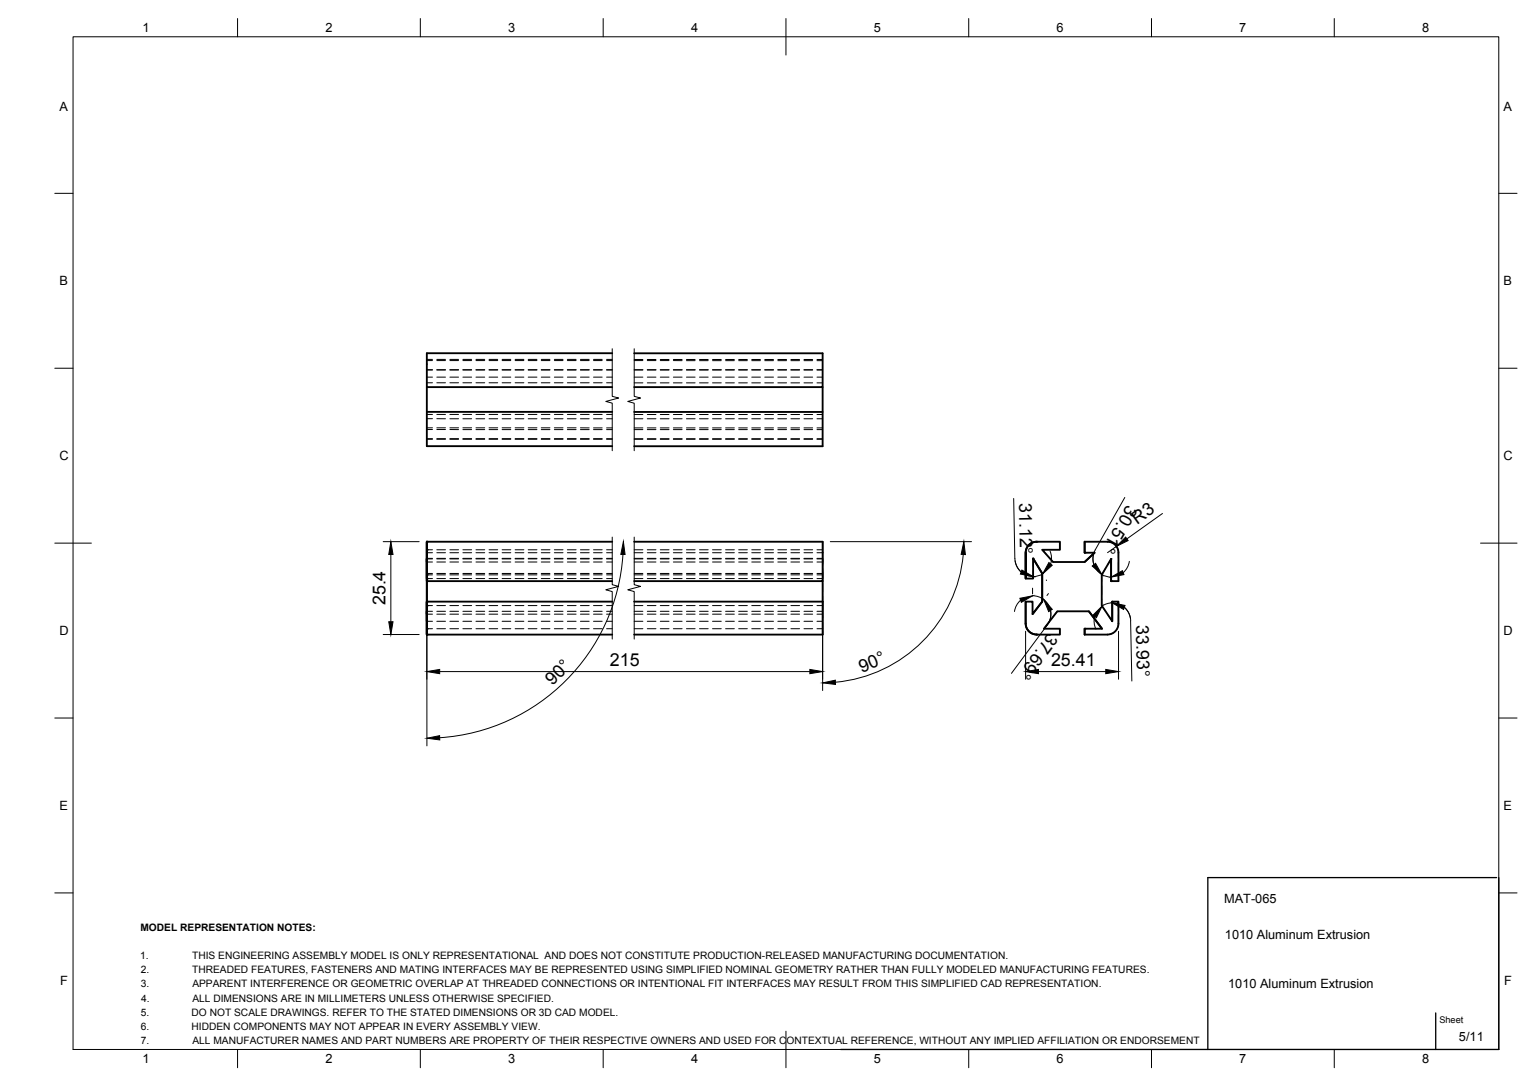
ISO-10303-21;
HEADER;
/* Generated by software containing ST-Developer
 * from STEP Tools, Inc. (www.steptools.com) 
 */

FILE_DESCRIPTION(
/* description */ (
'CAx-IF Rec.Pracs.---Representation and Presentation of Product Manufa
cturing Information (PMI)---4.0---2014-10-13'),
/* implementation_level */ '2;1');

FILE_NAME(
/* name */ '1010 Aluminum Extrusion.step',
/* time_stamp */ '2026-11-15T23:28:27-08:00',
/* author */ (''),
/* organization */ (''),
/* preprocessor_version */ 'ST-DEVELOPER v20.2',
/* originating_system */ 'Autodesk Translation Framework v15.17.0.0',
/* authorisation */ '');

FILE_SCHEMA (('AUTOMOTIVE_DESIGN { 1 0 10303 214 3 1 1 }'));
ENDSEC;

DATA;
#10=MECHANICAL_DESIGN_GEOMETRIC_PRESENTATION_REPRESENTATION('',(#194),#7756);
#176=SHAPE_REPRESENTATION_RELATIONSHIP('SRR','None',#7824,#185);
#185=ADVANCED_BREP_SHAPE_REPRESENTATION('',(#203),#7752);
#194=STYLED_ITEM('',(#7875),#203);
#203=MANIFOLD_SOLID_BREP('Body1',#4631);
#220=CYLINDRICAL_SURFACE('',#4850,0.003);
#221=CYLINDRICAL_SURFACE('',#4851,0.003);
#222=CYLINDRICAL_SURFACE('',#4852,0.003);
#223=CYLINDRICAL_SURFACE('',#4853,0.003);
#290=CIRCLE('',#4837,0.003);
#291=CIRCLE('',#4838,0.003);
#292=CIRCLE('',#4839,0.003);
#293=CIRCLE('',#4840,0.003);
#294=CIRCLE('',#4842,0.003);
#295=CIRCLE('',#4843,0.003);
#296=CIRCLE('',#4844,0.003);
#297=CIRCLE('',#4845,0.003);
#516=FACE_OUTER_BOUND('',#778,.T.);
#517=FACE_OUTER_BOUND('',#779,.T.);
#518=FACE_OUTER_BOUND('',#780,.T.);
#519=FACE_OUTER_BOUND('',#781,.T.);
#520=FACE_OUTER_BOUND('',#782,.T.);
#521=FACE_OUTER_BOUND('',#783,.T.);
#522=FACE_OUTER_BOUND('',#784,.T.);
#523=FACE_OUTER_BOUND('',#785,.T.);
#524=FACE_OUTER_BOUND('',#786,.T.);
#525=FACE_OUTER_BOUND('',#787,.T.);
#526=FACE_OUTER_BOUND('',#788,.T.);
#527=FACE_OUTER_BOUND('',#789,.T.);
#528=FACE_OUTER_BOUND('',#790,.T.);
#529=FACE_OUTER_BOUND('',#791,.T.);
#530=FACE_OUTER_BOUND('',#792,.T.);
#531=FACE_OUTER_BOUND('',#793,.T.);
#532=FACE_OUTER_BOUND('',#794,.T.);
#533=FACE_OUTER_BOUND('',#795,.T.);
#534=FACE_OUTER_BOUND('',#796,.T.);
#535=FACE_OUTER_BOUND('',#797,.T.);
#536=FACE_OUTER_BOUND('',#798,.T.);
#537=FACE_OUTER_BOUND('',#799,.T.);
#538=FACE_OUTER_BOUND('',#800,.T.);
#539=FACE_OUTER_BOUND('',#801,.T.);
#540=FACE_OUTER_BOUND('',#802,.T.);
#541=FACE_OUTER_BOUND('',#803,.T.);
#542=FACE_OUTER_BOUND('',#804,.T.);
#543=FACE_OUTER_BOUND('',#805,.T.);
#544=FACE_OUTER_BOUND('',#806,.T.);
#545=FACE_OUTER_BOUND('',#807,.T.);
#546=FACE_OUTER_BOUND('',#808,.T.);
#547=FACE_OUTER_BOUND('',#809,.T.);
#548=FACE_OUTER_BOUND('',#810,.T.);
#549=FACE_OUTER_BOUND('',#811,.T.);
#550=FACE_OUTER_BOUND('',#812,.T.);
#551=FACE_OUTER_BOUND('',#813,.T.);
#552=FACE_OUTER_BOUND('',#814,.T.);
#553=FACE_OUTER_BOUND('',#815,.T.);
#554=FACE_OUTER_BOUND('',#816,.T.);
#555=FACE_OUTER_BOUND('',#817,.T.);
#556=FACE_OUTER_BOUND('',#818,.T.);
#557=FACE_OUTER_BOUND('',#819,.T.);
#778=EDGE_LOOP('',(#3311,#3312,#3313,#3314));
#779=EDGE_LOOP('',(#3315,#3316,#3317,#3318));
#780=EDGE_LOOP('',(#3319,#3320,#3321,#3322));
#781=EDGE_LOOP('',(#3323,#3324,#3325,#3326));
#782=EDGE_LOOP('',(#3327,#3328,#3329,#3330,#3331,#3332,#3333,#3334,#3335,
#3336,#3337,#3338,#3339,#3340,#3341,#3342,#3343,#3344,#3345,#3346,#3347,
#3348,#3349,#3350,#3351,#3352,#3353,#3354,#3355,#3356,#3357,#3358,#3359,
#3360,#3361,#3362,#3363,#3364,#3365,#3366));
#783=EDGE_LOOP('',(#3367,#3368,#3369,#3370,#3371,#3372,#3373,#3374,#3375,
#3376,#3377,#3378,#3379,#3380,#3381,#3382,#3383,#3384,#3385,#3386,#3387,
#3388,#3389,#3390,#3391,#3392,#3393,#3394,#3395,#3396,#3397,#3398,#3399,
#3400,#3401,#3402,#3403,#3404,#3405,#3406));
#784=EDGE_LOOP('',(#3407,#3408,#3409,#3410));
#785=EDGE_LOOP('',(#3411,#3412,#3413,#3414));
#786=EDGE_LOOP('',(#3415,#3416,#3417,#3418));
#787=EDGE_LOOP('',(#3419,#3420,#3421,#3422));
#788=EDGE_LOOP('',(#3423,#3424,#3425,#3426));
#789=EDGE_LOOP('',(#3427,#3428,#3429,#3430));
#790=EDGE_LOOP('',(#3431,#3432,#3433,#3434));
#791=EDGE_LOOP('',(#3435,#3436,#3437,#3438));
#792=EDGE_LOOP('',(#3439,#3440,#3441,#3442));
#793=EDGE_LOOP('',(#3443,#3444,#3445,#3446));
#794=EDGE_LOOP('',(#3447,#3448,#3449,#3450));
#795=EDGE_LOOP('',(#3451,#3452,#3453,#3454));
#796=EDGE_LOOP('',(#3455,#3456,#3457,#3458));
#797=EDGE_LOOP('',(#3459,#3460,#3461,#3462));
#798=EDGE_LOOP('',(#3463,#3464,#3465,#3466));
#799=EDGE_LOOP('',(#3467,#3468,#3469,#3470));
#800=EDGE_LOOP('',(#3471,#3472,#3473,#3474));
#801=EDGE_LOOP('',(#3475,#3476,#3477,#3478));
#802=EDGE_LOOP('',(#3479,#3480,#3481,#3482));
#803=EDGE_LOOP('',(#3483,#3484,#3485,#3486));
#804=EDGE_LOOP('',(#3487,#3488,#3489,#3490));
#805=EDGE_LOOP('',(#3491,#3492,#3493,#3494));
#806=EDGE_LOOP('',(#3495,#3496,#3497,#3498));
#807=EDGE_LOOP('',(#3499,#3500,#3501,#3502));
#808=EDGE_LOOP('',(#3503,#3504,#3505,#3506));
#809=EDGE_LOOP('',(#3507,#3508,#3509,#3510));
#810=EDGE_LOOP('',(#3511,#3512,#3513,#3514));
#811=EDGE_LOOP('',(#3515,#3516,#3517,#3518));
#812=EDGE_LOOP('',(#3519,#3520,#3521,#3522));
#813=EDGE_LOOP('',(#3523,#3524,#3525,#3526));
#814=EDGE_LOOP('',(#3527,#3528,#3529,#3530));
#815=EDGE_LOOP('',(#3531,#3532,#3533,#3534));
#816=EDGE_LOOP('',(#3535,#3536,#3537,#3538));
#817=EDGE_LOOP('',(#3539,#3540,#3541,#3542));
#818=EDGE_LOOP('',(#3543,#3544,#3545,#3546));
#819=EDGE_LOOP('',(#3547,#3548,#3549,#3550));
#1125=LINE('',#6758,#1618);
#1126=LINE('',#6760,#1619);
#1127=LINE('',#6762,#1620);
#1128=LINE('',#6763,#1621);
#1129=LINE('',#6767,#1622);
#1130=LINE('',#6769,#1623);
#1131=LINE('',#6771,#1624);
#1132=LINE('',#6772,#1625);
#1133=LINE('',#6776,#1626);
#1134=LINE('',#6778,#1627);
#1135=LINE('',#6780,#1628);
#1136=LINE('',#6781,#1629);
#1137=LINE('',#6785,#1630);
#1138=LINE('',#6787,#1631);
#1139=LINE('',#6789,#1632);
#1140=LINE('',#6790,#1633);
#1141=LINE('',#6794,#1634);
#1142=LINE('',#6796,#1635);
#1143=LINE('',#6799,#1636);
#1144=LINE('',#6801,#1637);
#1145=LINE('',#6803,#1638);
#1146=LINE('',#6805,#1639);
#1147=LINE('',#6807,#1640);
#1148=LINE('',#6809,#1641);
#1149=LINE('',#6811,#1642);
#1150=LINE('',#6813,#1643);
#1151=LINE('',#6817,#1644);
#1152=LINE('',#6819,#1645);
#1153=LINE('',#6821,#1646);
#1154=LINE('',#6823,#1647);
#1155=LINE('',#6825,#1648);
#1156=LINE('',#6827,#1649);
#1157=LINE('',#6829,#1650);
#1158=LINE('',#6830,#1651);
#1159=LINE('',#6834,#1652);
#1160=LINE('',#6836,#1653);
#1161=LINE('',#6838,#1654);
#1162=LINE('',#6840,#1655);
#1163=LINE('',#6842,#1656);
#1164=LINE('',#6844,#1657);
#1165=LINE('',#6846,#1658);
#1166=LINE('',#6847,#1659);
#1167=LINE('',#6850,#1660);
#1168=LINE('',#6852,#1661);
#1169=LINE('',#6854,#1662);
#1170=LINE('',#6856,#1663);
#1171=LINE('',#6858,#1664);
#1172=LINE('',#6859,#1665);
#1173=LINE('',#6863,#1666);
#1174=LINE('',#6865,#1667);
#1175=LINE('',#6867,#1668);
#1176=LINE('',#6869,#1669);
#1177=LINE('',#6871,#1670);
#1178=LINE('',#6873,#1671);
#1179=LINE('',#6875,#1672);
#1180=LINE('',#6876,#1673);
#1181=LINE('',#6879,#1674);
#1182=LINE('',#6881,#1675);
#1183=LINE('',#6883,#1676);
#1184=LINE('',#6885,#1677);
#1185=LINE('',#6887,#1678);
#1186=LINE('',#6889,#1679);
#1187=LINE('',#6891,#1680);
#1188=LINE('',#6893,#1681);
#1189=LINE('',#6896,#1682);
#1190=LINE('',#6898,#1683);
#1191=LINE('',#6900,#1684);
#1192=LINE('',#6902,#1685);
#1193=LINE('',#6904,#1686);
#1194=LINE('',#6906,#1687);
#1195=LINE('',#6908,#1688);
#1196=LINE('',#6910,#1689);
#1197=LINE('',#6914,#1690);
#1198=LINE('',#6916,#1691);
#1199=LINE('',#6918,#1692);
#1200=LINE('',#6920,#1693);
#1201=LINE('',#6922,#1694);
#1202=LINE('',#6924,#1695);
#1203=LINE('',#6926,#1696);
#1204=LINE('',#6927,#1697);
#1205=LINE('',#6930,#1698);
#1206=LINE('',#6931,#1699);
#1207=LINE('',#6933,#1700);
#1208=LINE('',#6934,#1701);
#1209=LINE('',#6936,#1702);
#1210=LINE('',#6937,#1703);
#1211=LINE('',#6939,#1704);
#1212=LINE('',#6940,#1705);
#1213=LINE('',#6946,#1706);
#1214=LINE('',#6948,#1707);
#1215=LINE('',#6950,#1708);
#1216=LINE('',#6952,#1709);
#1217=LINE('',#6954,#1710);
#1218=LINE('',#6956,#1711);
#1219=LINE('',#6959,#1712);
#1220=LINE('',#6961,#1713);
#1221=LINE('',#6963,#1714);
#1222=LINE('',#6965,#1715);
#1223=LINE('',#6967,#1716);
#1224=LINE('',#6969,#1717);
#1225=LINE('',#6972,#1718);
#1226=LINE('',#6974,#1719);
#1227=LINE('',#6976,#1720);
#1228=LINE('',#6978,#1721);
#1229=LINE('',#6980,#1722);
#1230=LINE('',#6982,#1723);
#1231=LINE('',#6985,#1724);
#1232=LINE('',#6987,#1725);
#1233=LINE('',#6989,#1726);
#1234=LINE('',#6991,#1727);
#1235=LINE('',#6993,#1728);
#1236=LINE('',#6995,#1729);
#1618=VECTOR('',#5461,1.);
#1619=VECTOR('',#5462,1.);
#1620=VECTOR('',#5463,1.);
#1621=VECTOR('',#5464,1.);
#1622=VECTOR('',#5467,1.);
#1623=VECTOR('',#5468,1.);
#1624=VECTOR('',#5469,1.);
#1625=VECTOR('',#5470,1.);
#1626=VECTOR('',#5473,1.);
#1627=VECTOR('',#5474,1.);
#1628=VECTOR('',#5475,1.);
#1629=VECTOR('',#5476,1.);
#1630=VECTOR('',#5479,1.);
#1631=VECTOR('',#5480,1.);
#1632=VECTOR('',#5481,1.);
#1633=VECTOR('',#5482,1.);
#1634=VECTOR('',#5485,1.);
#1635=VECTOR('',#5486,1.);
#1636=VECTOR('',#5489,1.);
#1637=VECTOR('',#5490,1.);
#1638=VECTOR('',#5491,1.);
#1639=VECTOR('',#5492,1.);
#1640=VECTOR('',#5493,1.);
#1641=VECTOR('',#5494,1.);
#1642=VECTOR('',#5495,1.);
#1643=VECTOR('',#5496,1.);
#1644=VECTOR('',#5499,1.);
#1645=VECTOR('',#5500,1.);
#1646=VECTOR('',#5501,1.);
#1647=VECTOR('',#5502,1.);
#1648=VECTOR('',#5503,1.);
#1649=VECTOR('',#5504,1.);
#1650=VECTOR('',#5505,1.);
#1651=VECTOR('',#5506,1.);
#1652=VECTOR('',#5509,1.);
#1653=VECTOR('',#5510,1.);
#1654=VECTOR('',#5511,1.);
#1655=VECTOR('',#5512,1.);
#1656=VECTOR('',#5513,1.);
#1657=VECTOR('',#5514,1.);
#1658=VECTOR('',#5515,1.);
#1659=VECTOR('',#5516,1.);
#1660=VECTOR('',#5519,1.);
#1661=VECTOR('',#5520,1.);
#1662=VECTOR('',#5521,1.);
#1663=VECTOR('',#5522,1.);
#1664=VECTOR('',#5523,1.);
#1665=VECTOR('',#5524,1.);
#1666=VECTOR('',#5527,1.);
#1667=VECTOR('',#5528,1.);
#1668=VECTOR('',#5529,1.);
#1669=VECTOR('',#5530,1.);
#1670=VECTOR('',#5531,1.);
#1671=VECTOR('',#5532,1.);
#1672=VECTOR('',#5533,1.);
#1673=VECTOR('',#5534,1.);
#1674=VECTOR('',#5537,1.);
#1675=VECTOR('',#5538,1.);
#1676=VECTOR('',#5539,1.);
#1677=VECTOR('',#5540,1.);
#1678=VECTOR('',#5541,1.);
#1679=VECTOR('',#5542,1.);
#1680=VECTOR('',#5543,1.);
#1681=VECTOR('',#5544,1.);
#1682=VECTOR('',#5547,1.);
#1683=VECTOR('',#5548,1.);
#1684=VECTOR('',#5549,1.);
#1685=VECTOR('',#5550,1.);
#1686=VECTOR('',#5551,1.);
#1687=VECTOR('',#5552,1.);
#1688=VECTOR('',#5553,1.);
#1689=VECTOR('',#5554,1.);
#1690=VECTOR('',#5557,1.);
#1691=VECTOR('',#5558,1.);
#1692=VECTOR('',#5559,1.);
#1693=VECTOR('',#5560,1.);
#1694=VECTOR('',#5561,1.);
#1695=VECTOR('',#5562,1.);
#1696=VECTOR('',#5563,1.);
#1697=VECTOR('',#5564,1.);
#1698=VECTOR('',#5569,1.);
#1699=VECTOR('',#5570,1.);
#1700=VECTOR('',#5573,1.);
#1701=VECTOR('',#5574,1.);
#1702=VECTOR('',#5577,1.);
#1703=VECTOR('',#5578,1.);
#1704=VECTOR('',#5581,1.);
#1705=VECTOR('',#5582,1.);
#1706=VECTOR('',#5593,1.);
#1707=VECTOR('',#5596,1.);
#1708=VECTOR('',#5599,1.);
#1709=VECTOR('',#5602,1.);
#1710=VECTOR('',#5605,1.);
#1711=VECTOR('',#5608,1.);
#1712=VECTOR('',#5613,1.);
#1713=VECTOR('',#5616,1.);
#1714=VECTOR('',#5619,1.);
#1715=VECTOR('',#5622,1.);
#1716=VECTOR('',#5625,1.);
#1717=VECTOR('',#5628,1.);
#1718=VECTOR('',#5633,1.);
#1719=VECTOR('',#5636,1.);
#1720=VECTOR('',#5639,1.);
#1721=VECTOR('',#5642,1.);
#1722=VECTOR('',#5645,1.);
#1723=VECTOR('',#5648,1.);
#1724=VECTOR('',#5653,1.);
#1725=VECTOR('',#5656,1.);
#1726=VECTOR('',#5659,1.);
#1727=VECTOR('',#5662,1.);
#1728=VECTOR('',#5665,1.);
#1729=VECTOR('',#5668,1.);
#2084=VERTEX_POINT('',#6756);
#2085=VERTEX_POINT('',#6757);
#2086=VERTEX_POINT('',#6759);
#2087=VERTEX_POINT('',#6761);
#2088=VERTEX_POINT('',#6765);
#2089=VERTEX_POINT('',#6766);
#2090=VERTEX_POINT('',#6768);
#2091=VERTEX_POINT('',#6770);
#2092=VERTEX_POINT('',#6774);
#2093=VERTEX_POINT('',#6775);
#2094=VERTEX_POINT('',#6777);
#2095=VERTEX_POINT('',#6779);
#2096=VERTEX_POINT('',#6783);
#2097=VERTEX_POINT('',#6784);
#2098=VERTEX_POINT('',#6786);
#2099=VERTEX_POINT('',#6788);
#2100=VERTEX_POINT('',#6792);
#2101=VERTEX_POINT('',#6793);
#2102=VERTEX_POINT('',#6795);
#2103=VERTEX_POINT('',#6798);
#2104=VERTEX_POINT('',#6800);
#2105=VERTEX_POINT('',#6802);
#2106=VERTEX_POINT('',#6804);
#2107=VERTEX_POINT('',#6806);
#2108=VERTEX_POINT('',#6808);
#2109=VERTEX_POINT('',#6810);
#2110=VERTEX_POINT('',#6812);
#2111=VERTEX_POINT('',#6814);
#2112=VERTEX_POINT('',#6816);
#2113=VERTEX_POINT('',#6818);
#2114=VERTEX_POINT('',#6820);
#2115=VERTEX_POINT('',#6822);
#2116=VERTEX_POINT('',#6824);
#2117=VERTEX_POINT('',#6826);
#2118=VERTEX_POINT('',#6828);
#2119=VERTEX_POINT('',#6831);
#2120=VERTEX_POINT('',#6833);
#2121=VERTEX_POINT('',#6835);
#2122=VERTEX_POINT('',#6837);
#2123=VERTEX_POINT('',#6839);
#2124=VERTEX_POINT('',#6841);
#2125=VERTEX_POINT('',#6843);
#2126=VERTEX_POINT('',#6845);
#2127=VERTEX_POINT('',#6849);
#2128=VERTEX_POINT('',#6851);
#2129=VERTEX_POINT('',#6853);
#2130=VERTEX_POINT('',#6855);
#2131=VERTEX_POINT('',#6857);
#2132=VERTEX_POINT('',#6861);
#2133=VERTEX_POINT('',#6862);
#2134=VERTEX_POINT('',#6864);
#2135=VERTEX_POINT('',#6866);
#2136=VERTEX_POINT('',#6868);
#2137=VERTEX_POINT('',#6870);
#2138=VERTEX_POINT('',#6872);
#2139=VERTEX_POINT('',#6874);
#2140=VERTEX_POINT('',#6878);
#2141=VERTEX_POINT('',#6880);
#2142=VERTEX_POINT('',#6882);
#2143=VERTEX_POINT('',#6884);
#2144=VERTEX_POINT('',#6886);
#2145=VERTEX_POINT('',#6888);
#2146=VERTEX_POINT('',#6890);
#2147=VERTEX_POINT('',#6892);
#2148=VERTEX_POINT('',#6895);
#2149=VERTEX_POINT('',#6897);
#2150=VERTEX_POINT('',#6899);
#2151=VERTEX_POINT('',#6901);
#2152=VERTEX_POINT('',#6903);
#2153=VERTEX_POINT('',#6905);
#2154=VERTEX_POINT('',#6907);
#2155=VERTEX_POINT('',#6909);
#2156=VERTEX_POINT('',#6911);
#2157=VERTEX_POINT('',#6913);
#2158=VERTEX_POINT('',#6915);
#2159=VERTEX_POINT('',#6917);
#2160=VERTEX_POINT('',#6919);
#2161=VERTEX_POINT('',#6921);
#2162=VERTEX_POINT('',#6923);
#2163=VERTEX_POINT('',#6925);
#2539=EDGE_CURVE('',#2084,#2085,#1125,.T.);
#2540=EDGE_CURVE('',#2084,#2086,#1126,.T.);
#2541=EDGE_CURVE('',#2086,#2087,#1127,.T.);
#2542=EDGE_CURVE('',#2087,#2085,#1128,.T.);
#2543=EDGE_CURVE('',#2088,#2089,#1129,.T.);
#2544=EDGE_CURVE('',#2088,#2090,#1130,.T.);
#2545=EDGE_CURVE('',#2090,#2091,#1131,.F.);
#2546=EDGE_CURVE('',#2089,#2091,#1132,.T.);
#2547=EDGE_CURVE('',#2092,#2093,#1133,.T.);
#2548=EDGE_CURVE('',#2092,#2094,#1134,.T.);
#2549=EDGE_CURVE('',#2094,#2095,#1135,.F.);
#2550=EDGE_CURVE('',#2093,#2095,#1136,.T.);
#2551=EDGE_CURVE('',#2096,#2097,#1137,.T.);
#2552=EDGE_CURVE('',#2096,#2098,#1138,.T.);
#2553=EDGE_CURVE('',#2098,#2099,#1139,.T.);
#2554=EDGE_CURVE('',#2099,#2097,#1140,.T.);
#2555=EDGE_CURVE('',#2100,#2101,#1141,.T.);
#2556=EDGE_CURVE('',#2102,#2100,#1142,.T.);
#2557=EDGE_CURVE('',#2102,#2087,#290,.T.);
#2558=EDGE_CURVE('',#2103,#2086,#1143,.T.);
#2559=EDGE_CURVE('',#2104,#2103,#1144,.T.);
#2560=EDGE_CURVE('',#2105,#2104,#1145,.T.);
#2561=EDGE_CURVE('',#2106,#2105,#1146,.T.);
#2562=EDGE_CURVE('',#2107,#2106,#1147,.T.);
#2563=EDGE_CURVE('',#2108,#2107,#1148,.T.);
#2564=EDGE_CURVE('',#2109,#2108,#1149,.T.);
#2565=EDGE_CURVE('',#2110,#2109,#1150,.T.);
#2566=EDGE_CURVE('',#2110,#2111,#291,.T.);
#2567=EDGE_CURVE('',#2111,#2112,#1151,.T.);
#2568=EDGE_CURVE('',#2113,#2112,#1152,.T.);
#2569=EDGE_CURVE('',#2114,#2113,#1153,.T.);
#2570=EDGE_CURVE('',#2115,#2114,#1154,.T.);
#2571=EDGE_CURVE('',#2116,#2115,#1155,.T.);
#2572=EDGE_CURVE('',#2117,#2116,#1156,.T.);
#2573=EDGE_CURVE('',#2118,#2117,#1157,.T.);
#2574=EDGE_CURVE('',#2089,#2118,#1158,.T.);
#2575=EDGE_CURVE('',#2091,#2119,#292,.T.);
#2576=EDGE_CURVE('',#2119,#2120,#1159,.T.);
#2577=EDGE_CURVE('',#2120,#2121,#1160,.T.);
#2578=EDGE_CURVE('',#2121,#2122,#1161,.T.);
#2579=EDGE_CURVE('',#2122,#2123,#1162,.T.);
#2580=EDGE_CURVE('',#2123,#2124,#1163,.T.);
#2581=EDGE_CURVE('',#2124,#2125,#1164,.T.);
#2582=EDGE_CURVE('',#2125,#2126,#1165,.T.);
#2583=EDGE_CURVE('',#2126,#2093,#1166,.T.);
#2584=EDGE_CURVE('',#2095,#2099,#293,.T.);
#2585=EDGE_CURVE('',#2127,#2098,#1167,.T.);
#2586=EDGE_CURVE('',#2128,#2127,#1168,.T.);
#2587=EDGE_CURVE('',#2129,#2128,#1169,.T.);
#2588=EDGE_CURVE('',#2130,#2129,#1170,.T.);
#2589=EDGE_CURVE('',#2131,#2130,#1171,.T.);
#2590=EDGE_CURVE('',#2101,#2131,#1172,.T.);
#2591=EDGE_CURVE('',#2132,#2133,#1173,.T.);
#2592=EDGE_CURVE('',#2133,#2134,#1174,.T.);
#2593=EDGE_CURVE('',#2134,#2135,#1175,.T.);
#2594=EDGE_CURVE('',#2135,#2136,#1176,.T.);
#2595=EDGE_CURVE('',#2136,#2137,#1177,.T.);
#2596=EDGE_CURVE('',#2137,#2138,#1178,.T.);
#2597=EDGE_CURVE('',#2138,#2139,#1179,.T.);
#2598=EDGE_CURVE('',#2139,#2096,#1180,.T.);
#2599=EDGE_CURVE('',#2097,#2094,#294,.F.);
#2600=EDGE_CURVE('',#2140,#2092,#1181,.T.);
#2601=EDGE_CURVE('',#2141,#2140,#1182,.T.);
#2602=EDGE_CURVE('',#2142,#2141,#1183,.T.);
#2603=EDGE_CURVE('',#2143,#2142,#1184,.T.);
#2604=EDGE_CURVE('',#2144,#2143,#1185,.T.);
#2605=EDGE_CURVE('',#2145,#2144,#1186,.T.);
#2606=EDGE_CURVE('',#2146,#2145,#1187,.T.);
#2607=EDGE_CURVE('',#2147,#2146,#1188,.T.);
#2608=EDGE_CURVE('',#2147,#2090,#295,.F.);
#2609=EDGE_CURVE('',#2088,#2148,#1189,.T.);
#2610=EDGE_CURVE('',#2148,#2149,#1190,.T.);
#2611=EDGE_CURVE('',#2149,#2150,#1191,.T.);
#2612=EDGE_CURVE('',#2150,#2151,#1192,.T.);
#2613=EDGE_CURVE('',#2151,#2152,#1193,.T.);
#2614=EDGE_CURVE('',#2152,#2153,#1194,.T.);
#2615=EDGE_CURVE('',#2153,#2154,#1195,.T.);
#2616=EDGE_CURVE('',#2155,#2154,#1196,.T.);
#2617=EDGE_CURVE('',#2155,#2156,#296,.F.);
#2618=EDGE_CURVE('',#2156,#2157,#1197,.T.);
#2619=EDGE_CURVE('',#2157,#2158,#1198,.T.);
#2620=EDGE_CURVE('',#2158,#2159,#1199,.T.);
#2621=EDGE_CURVE('',#2159,#2160,#1200,.T.);
#2622=EDGE_CURVE('',#2160,#2161,#1201,.T.);
#2623=EDGE_CURVE('',#2161,#2162,#1202,.T.);
#2624=EDGE_CURVE('',#2162,#2163,#1203,.T.);
#2625=EDGE_CURVE('',#2163,#2084,#1204,.T.);
#2626=EDGE_CURVE('',#2085,#2132,#297,.F.);
#2627=EDGE_CURVE('',#2157,#2109,#1205,.T.);
#2628=EDGE_CURVE('',#2156,#2110,#1206,.F.);
#2629=EDGE_CURVE('',#2154,#2112,#1207,.T.);
#2630=EDGE_CURVE('',#2111,#2155,#1208,.T.);
#2631=EDGE_CURVE('',#2146,#2120,#1209,.T.);
#2632=EDGE_CURVE('',#2119,#2147,#1210,.T.);
#2633=EDGE_CURVE('',#2133,#2100,#1211,.T.);
#2634=EDGE_CURVE('',#2132,#2102,#1212,.F.);
#2635=EDGE_CURVE('',#2158,#2108,#1213,.T.);
#2636=EDGE_CURVE('',#2159,#2107,#1214,.T.);
#2637=EDGE_CURVE('',#2160,#2106,#1215,.T.);
#2638=EDGE_CURVE('',#2161,#2105,#1216,.T.);
#2639=EDGE_CURVE('',#2162,#2104,#1217,.T.);
#2640=EDGE_CURVE('',#2163,#2103,#1218,.T.);
#2641=EDGE_CURVE('',#2148,#2118,#1219,.T.);
#2642=EDGE_CURVE('',#2149,#2117,#1220,.T.);
#2643=EDGE_CURVE('',#2150,#2116,#1221,.T.);
#2644=EDGE_CURVE('',#2151,#2115,#1222,.T.);
#2645=EDGE_CURVE('',#2152,#2114,#1223,.T.);
#2646=EDGE_CURVE('',#2153,#2113,#1224,.T.);
#2647=EDGE_CURVE('',#2145,#2121,#1225,.T.);
#2648=EDGE_CURVE('',#2140,#2126,#1226,.T.);
#2649=EDGE_CURVE('',#2141,#2125,#1227,.T.);
#2650=EDGE_CURVE('',#2142,#2124,#1228,.T.);
#2651=EDGE_CURVE('',#2143,#2123,#1229,.T.);
#2652=EDGE_CURVE('',#2144,#2122,#1230,.T.);
#2653=EDGE_CURVE('',#2134,#2101,#1231,.T.);
#2654=EDGE_CURVE('',#2135,#2131,#1232,.T.);
#2655=EDGE_CURVE('',#2136,#2130,#1233,.T.);
#2656=EDGE_CURVE('',#2137,#2129,#1234,.T.);
#2657=EDGE_CURVE('',#2138,#2128,#1235,.T.);
#2658=EDGE_CURVE('',#2139,#2127,#1236,.T.);
#3311=ORIENTED_EDGE('',*,*,#2539,.F.);
#3312=ORIENTED_EDGE('',*,*,#2540,.T.);
#3313=ORIENTED_EDGE('',*,*,#2541,.T.);
#3314=ORIENTED_EDGE('',*,*,#2542,.T.);
#3315=ORIENTED_EDGE('',*,*,#2543,.F.);
#3316=ORIENTED_EDGE('',*,*,#2544,.T.);
#3317=ORIENTED_EDGE('',*,*,#2545,.T.);
#3318=ORIENTED_EDGE('',*,*,#2546,.F.);
#3319=ORIENTED_EDGE('',*,*,#2547,.F.);
#3320=ORIENTED_EDGE('',*,*,#2548,.T.);
#3321=ORIENTED_EDGE('',*,*,#2549,.T.);
#3322=ORIENTED_EDGE('',*,*,#2550,.F.);
#3323=ORIENTED_EDGE('',*,*,#2551,.F.);
#3324=ORIENTED_EDGE('',*,*,#2552,.T.);
#3325=ORIENTED_EDGE('',*,*,#2553,.T.);
#3326=ORIENTED_EDGE('',*,*,#2554,.T.);
#3327=ORIENTED_EDGE('',*,*,#2555,.F.);
#3328=ORIENTED_EDGE('',*,*,#2556,.F.);
#3329=ORIENTED_EDGE('',*,*,#2557,.T.);
#3330=ORIENTED_EDGE('',*,*,#2541,.F.);
#3331=ORIENTED_EDGE('',*,*,#2558,.F.);
#3332=ORIENTED_EDGE('',*,*,#2559,.F.);
#3333=ORIENTED_EDGE('',*,*,#2560,.F.);
#3334=ORIENTED_EDGE('',*,*,#2561,.F.);
#3335=ORIENTED_EDGE('',*,*,#2562,.F.);
#3336=ORIENTED_EDGE('',*,*,#2563,.F.);
#3337=ORIENTED_EDGE('',*,*,#2564,.F.);
#3338=ORIENTED_EDGE('',*,*,#2565,.F.);
#3339=ORIENTED_EDGE('',*,*,#2566,.T.);
#3340=ORIENTED_EDGE('',*,*,#2567,.T.);
#3341=ORIENTED_EDGE('',*,*,#2568,.F.);
#3342=ORIENTED_EDGE('',*,*,#2569,.F.);
#3343=ORIENTED_EDGE('',*,*,#2570,.F.);
#3344=ORIENTED_EDGE('',*,*,#2571,.F.);
#3345=ORIENTED_EDGE('',*,*,#2572,.F.);
#3346=ORIENTED_EDGE('',*,*,#2573,.F.);
#3347=ORIENTED_EDGE('',*,*,#2574,.F.);
#3348=ORIENTED_EDGE('',*,*,#2546,.T.);
#3349=ORIENTED_EDGE('',*,*,#2575,.T.);
#3350=ORIENTED_EDGE('',*,*,#2576,.T.);
#3351=ORIENTED_EDGE('',*,*,#2577,.T.);
#3352=ORIENTED_EDGE('',*,*,#2578,.T.);
#3353=ORIENTED_EDGE('',*,*,#2579,.T.);
#3354=ORIENTED_EDGE('',*,*,#2580,.T.);
#3355=ORIENTED_EDGE('',*,*,#2581,.T.);
#3356=ORIENTED_EDGE('',*,*,#2582,.T.);
#3357=ORIENTED_EDGE('',*,*,#2583,.T.);
#3358=ORIENTED_EDGE('',*,*,#2550,.T.);
#3359=ORIENTED_EDGE('',*,*,#2584,.T.);
#3360=ORIENTED_EDGE('',*,*,#2553,.F.);
#3361=ORIENTED_EDGE('',*,*,#2585,.F.);
#3362=ORIENTED_EDGE('',*,*,#2586,.F.);
#3363=ORIENTED_EDGE('',*,*,#2587,.F.);
#3364=ORIENTED_EDGE('',*,*,#2588,.F.);
#3365=ORIENTED_EDGE('',*,*,#2589,.F.);
#3366=ORIENTED_EDGE('',*,*,#2590,.F.);
#3367=ORIENTED_EDGE('',*,*,#2591,.T.);
#3368=ORIENTED_EDGE('',*,*,#2592,.T.);
#3369=ORIENTED_EDGE('',*,*,#2593,.T.);
#3370=ORIENTED_EDGE('',*,*,#2594,.T.);
#3371=ORIENTED_EDGE('',*,*,#2595,.T.);
#3372=ORIENTED_EDGE('',*,*,#2596,.T.);
#3373=ORIENTED_EDGE('',*,*,#2597,.T.);
#3374=ORIENTED_EDGE('',*,*,#2598,.T.);
#3375=ORIENTED_EDGE('',*,*,#2551,.T.);
#3376=ORIENTED_EDGE('',*,*,#2599,.T.);
#3377=ORIENTED_EDGE('',*,*,#2548,.F.);
#3378=ORIENTED_EDGE('',*,*,#2600,.F.);
#3379=ORIENTED_EDGE('',*,*,#2601,.F.);
#3380=ORIENTED_EDGE('',*,*,#2602,.F.);
#3381=ORIENTED_EDGE('',*,*,#2603,.F.);
#3382=ORIENTED_EDGE('',*,*,#2604,.F.);
#3383=ORIENTED_EDGE('',*,*,#2605,.F.);
#3384=ORIENTED_EDGE('',*,*,#2606,.F.);
#3385=ORIENTED_EDGE('',*,*,#2607,.F.);
#3386=ORIENTED_EDGE('',*,*,#2608,.T.);
#3387=ORIENTED_EDGE('',*,*,#2544,.F.);
#3388=ORIENTED_EDGE('',*,*,#2609,.T.);
#3389=ORIENTED_EDGE('',*,*,#2610,.T.);
#3390=ORIENTED_EDGE('',*,*,#2611,.T.);
#3391=ORIENTED_EDGE('',*,*,#2612,.T.);
#3392=ORIENTED_EDGE('',*,*,#2613,.T.);
#3393=ORIENTED_EDGE('',*,*,#2614,.T.);
#3394=ORIENTED_EDGE('',*,*,#2615,.T.);
#3395=ORIENTED_EDGE('',*,*,#2616,.F.);
#3396=ORIENTED_EDGE('',*,*,#2617,.T.);
#3397=ORIENTED_EDGE('',*,*,#2618,.T.);
#3398=ORIENTED_EDGE('',*,*,#2619,.T.);
#3399=ORIENTED_EDGE('',*,*,#2620,.T.);
#3400=ORIENTED_EDGE('',*,*,#2621,.T.);
#3401=ORIENTED_EDGE('',*,*,#2622,.T.);
#3402=ORIENTED_EDGE('',*,*,#2623,.T.);
#3403=ORIENTED_EDGE('',*,*,#2624,.T.);
#3404=ORIENTED_EDGE('',*,*,#2625,.T.);
#3405=ORIENTED_EDGE('',*,*,#2539,.T.);
#3406=ORIENTED_EDGE('',*,*,#2626,.T.);
#3407=ORIENTED_EDGE('',*,*,#2627,.F.);
#3408=ORIENTED_EDGE('',*,*,#2618,.F.);
#3409=ORIENTED_EDGE('',*,*,#2628,.T.);
#3410=ORIENTED_EDGE('',*,*,#2565,.T.);
#3411=ORIENTED_EDGE('',*,*,#2616,.T.);
#3412=ORIENTED_EDGE('',*,*,#2629,.T.);
#3413=ORIENTED_EDGE('',*,*,#2567,.F.);
#3414=ORIENTED_EDGE('',*,*,#2630,.T.);
#3415=ORIENTED_EDGE('',*,*,#2607,.T.);
#3416=ORIENTED_EDGE('',*,*,#2631,.T.);
#3417=ORIENTED_EDGE('',*,*,#2576,.F.);
#3418=ORIENTED_EDGE('',*,*,#2632,.T.);
#3419=ORIENTED_EDGE('',*,*,#2633,.F.);
#3420=ORIENTED_EDGE('',*,*,#2591,.F.);
#3421=ORIENTED_EDGE('',*,*,#2634,.T.);
#3422=ORIENTED_EDGE('',*,*,#2556,.T.);
#3423=ORIENTED_EDGE('',*,*,#2566,.F.);
#3424=ORIENTED_EDGE('',*,*,#2628,.F.);
#3425=ORIENTED_EDGE('',*,*,#2617,.F.);
#3426=ORIENTED_EDGE('',*,*,#2630,.F.);
#3427=ORIENTED_EDGE('',*,*,#2575,.F.);
#3428=ORIENTED_EDGE('',*,*,#2545,.F.);
#3429=ORIENTED_EDGE('',*,*,#2608,.F.);
#3430=ORIENTED_EDGE('',*,*,#2632,.F.);
#3431=ORIENTED_EDGE('',*,*,#2584,.F.);
#3432=ORIENTED_EDGE('',*,*,#2549,.F.);
#3433=ORIENTED_EDGE('',*,*,#2599,.F.);
#3434=ORIENTED_EDGE('',*,*,#2554,.F.);
#3435=ORIENTED_EDGE('',*,*,#2557,.F.);
#3436=ORIENTED_EDGE('',*,*,#2634,.F.);
#3437=ORIENTED_EDGE('',*,*,#2626,.F.);
#3438=ORIENTED_EDGE('',*,*,#2542,.F.);
#3439=ORIENTED_EDGE('',*,*,#2627,.T.);
#3440=ORIENTED_EDGE('',*,*,#2564,.T.);
#3441=ORIENTED_EDGE('',*,*,#2635,.F.);
#3442=ORIENTED_EDGE('',*,*,#2619,.F.);
#3443=ORIENTED_EDGE('',*,*,#2635,.T.);
#3444=ORIENTED_EDGE('',*,*,#2563,.T.);
#3445=ORIENTED_EDGE('',*,*,#2636,.F.);
#3446=ORIENTED_EDGE('',*,*,#2620,.F.);
#3447=ORIENTED_EDGE('',*,*,#2636,.T.);
#3448=ORIENTED_EDGE('',*,*,#2562,.T.);
#3449=ORIENTED_EDGE('',*,*,#2637,.F.);
#3450=ORIENTED_EDGE('',*,*,#2621,.F.);
#3451=ORIENTED_EDGE('',*,*,#2637,.T.);
#3452=ORIENTED_EDGE('',*,*,#2561,.T.);
#3453=ORIENTED_EDGE('',*,*,#2638,.F.);
#3454=ORIENTED_EDGE('',*,*,#2622,.F.);
#3455=ORIENTED_EDGE('',*,*,#2638,.T.);
#3456=ORIENTED_EDGE('',*,*,#2560,.T.);
#3457=ORIENTED_EDGE('',*,*,#2639,.F.);
#3458=ORIENTED_EDGE('',*,*,#2623,.F.);
#3459=ORIENTED_EDGE('',*,*,#2639,.T.);
#3460=ORIENTED_EDGE('',*,*,#2559,.T.);
#3461=ORIENTED_EDGE('',*,*,#2640,.F.);
#3462=ORIENTED_EDGE('',*,*,#2624,.F.);
#3463=ORIENTED_EDGE('',*,*,#2640,.T.);
#3464=ORIENTED_EDGE('',*,*,#2558,.T.);
#3465=ORIENTED_EDGE('',*,*,#2540,.F.);
#3466=ORIENTED_EDGE('',*,*,#2625,.F.);
#3467=ORIENTED_EDGE('',*,*,#2543,.T.);
#3468=ORIENTED_EDGE('',*,*,#2574,.T.);
#3469=ORIENTED_EDGE('',*,*,#2641,.F.);
#3470=ORIENTED_EDGE('',*,*,#2609,.F.);
#3471=ORIENTED_EDGE('',*,*,#2641,.T.);
#3472=ORIENTED_EDGE('',*,*,#2573,.T.);
#3473=ORIENTED_EDGE('',*,*,#2642,.F.);
#3474=ORIENTED_EDGE('',*,*,#2610,.F.);
#3475=ORIENTED_EDGE('',*,*,#2642,.T.);
#3476=ORIENTED_EDGE('',*,*,#2572,.T.);
#3477=ORIENTED_EDGE('',*,*,#2643,.F.);
#3478=ORIENTED_EDGE('',*,*,#2611,.F.);
#3479=ORIENTED_EDGE('',*,*,#2643,.T.);
#3480=ORIENTED_EDGE('',*,*,#2571,.T.);
#3481=ORIENTED_EDGE('',*,*,#2644,.F.);
#3482=ORIENTED_EDGE('',*,*,#2612,.F.);
#3483=ORIENTED_EDGE('',*,*,#2644,.T.);
#3484=ORIENTED_EDGE('',*,*,#2570,.T.);
#3485=ORIENTED_EDGE('',*,*,#2645,.F.);
#3486=ORIENTED_EDGE('',*,*,#2613,.F.);
#3487=ORIENTED_EDGE('',*,*,#2645,.T.);
#3488=ORIENTED_EDGE('',*,*,#2569,.T.);
#3489=ORIENTED_EDGE('',*,*,#2646,.F.);
#3490=ORIENTED_EDGE('',*,*,#2614,.F.);
#3491=ORIENTED_EDGE('',*,*,#2646,.T.);
#3492=ORIENTED_EDGE('',*,*,#2568,.T.);
#3493=ORIENTED_EDGE('',*,*,#2629,.F.);
#3494=ORIENTED_EDGE('',*,*,#2615,.F.);
#3495=ORIENTED_EDGE('',*,*,#2606,.T.);
#3496=ORIENTED_EDGE('',*,*,#2647,.T.);
#3497=ORIENTED_EDGE('',*,*,#2577,.F.);
#3498=ORIENTED_EDGE('',*,*,#2631,.F.);
#3499=ORIENTED_EDGE('',*,*,#2600,.T.);
#3500=ORIENTED_EDGE('',*,*,#2547,.T.);
#3501=ORIENTED_EDGE('',*,*,#2583,.F.);
#3502=ORIENTED_EDGE('',*,*,#2648,.F.);
#3503=ORIENTED_EDGE('',*,*,#2601,.T.);
#3504=ORIENTED_EDGE('',*,*,#2648,.T.);
#3505=ORIENTED_EDGE('',*,*,#2582,.F.);
#3506=ORIENTED_EDGE('',*,*,#2649,.F.);
#3507=ORIENTED_EDGE('',*,*,#2602,.T.);
#3508=ORIENTED_EDGE('',*,*,#2649,.T.);
#3509=ORIENTED_EDGE('',*,*,#2581,.F.);
#3510=ORIENTED_EDGE('',*,*,#2650,.F.);
#3511=ORIENTED_EDGE('',*,*,#2603,.T.);
#3512=ORIENTED_EDGE('',*,*,#2650,.T.);
#3513=ORIENTED_EDGE('',*,*,#2580,.F.);
#3514=ORIENTED_EDGE('',*,*,#2651,.F.);
#3515=ORIENTED_EDGE('',*,*,#2604,.T.);
#3516=ORIENTED_EDGE('',*,*,#2651,.T.);
#3517=ORIENTED_EDGE('',*,*,#2579,.F.);
#3518=ORIENTED_EDGE('',*,*,#2652,.F.);
#3519=ORIENTED_EDGE('',*,*,#2605,.T.);
#3520=ORIENTED_EDGE('',*,*,#2652,.T.);
#3521=ORIENTED_EDGE('',*,*,#2578,.F.);
#3522=ORIENTED_EDGE('',*,*,#2647,.F.);
#3523=ORIENTED_EDGE('',*,*,#2633,.T.);
#3524=ORIENTED_EDGE('',*,*,#2555,.T.);
#3525=ORIENTED_EDGE('',*,*,#2653,.F.);
#3526=ORIENTED_EDGE('',*,*,#2592,.F.);
#3527=ORIENTED_EDGE('',*,*,#2653,.T.);
#3528=ORIENTED_EDGE('',*,*,#2590,.T.);
#3529=ORIENTED_EDGE('',*,*,#2654,.F.);
#3530=ORIENTED_EDGE('',*,*,#2593,.F.);
#3531=ORIENTED_EDGE('',*,*,#2654,.T.);
#3532=ORIENTED_EDGE('',*,*,#2589,.T.);
#3533=ORIENTED_EDGE('',*,*,#2655,.F.);
#3534=ORIENTED_EDGE('',*,*,#2594,.F.);
#3535=ORIENTED_EDGE('',*,*,#2655,.T.);
#3536=ORIENTED_EDGE('',*,*,#2588,.T.);
#3537=ORIENTED_EDGE('',*,*,#2656,.F.);
#3538=ORIENTED_EDGE('',*,*,#2595,.F.);
#3539=ORIENTED_EDGE('',*,*,#2656,.T.);
#3540=ORIENTED_EDGE('',*,*,#2587,.T.);
#3541=ORIENTED_EDGE('',*,*,#2657,.F.);
#3542=ORIENTED_EDGE('',*,*,#2596,.F.);
#3543=ORIENTED_EDGE('',*,*,#2657,.T.);
#3544=ORIENTED_EDGE('',*,*,#2586,.T.);
#3545=ORIENTED_EDGE('',*,*,#2658,.F.);
#3546=ORIENTED_EDGE('',*,*,#2597,.F.);
#3547=ORIENTED_EDGE('',*,*,#2658,.T.);
#3548=ORIENTED_EDGE('',*,*,#2585,.T.);
#3549=ORIENTED_EDGE('',*,*,#2552,.F.);
#3550=ORIENTED_EDGE('',*,*,#2598,.F.);
#4270=PLANE('',#4832);
#4271=PLANE('',#4833);
#4272=PLANE('',#4834);
#4273=PLANE('',#4835);
#4274=PLANE('',#4836);
#4275=PLANE('',#4841);
#4276=PLANE('',#4846);
#4277=PLANE('',#4847);
#4278=PLANE('',#4848);
#4279=PLANE('',#4849);
#4280=PLANE('',#4854);
#4281=PLANE('',#4855);
#4282=PLANE('',#4856);
#4283=PLANE('',#4857);
#4284=PLANE('',#4858);
#4285=PLANE('',#4859);
#4286=PLANE('',#4860);
#4287=PLANE('',#4861);
#4288=PLANE('',#4862);
#4289=PLANE('',#4863);
#4290=PLANE('',#4864);
#4291=PLANE('',#4865);
#4292=PLANE('',#4866);
#4293=PLANE('',#4867);
#4294=PLANE('',#4868);
#4295=PLANE('',#4869);
#4296=PLANE('',#4870);
#4297=PLANE('',#4871);
#4298=PLANE('',#4872);
#4299=PLANE('',#4873);
#4300=PLANE('',#4874);
#4301=PLANE('',#4875);
#4302=PLANE('',#4876);
#4303=PLANE('',#4877);
#4304=PLANE('',#4878);
#4305=PLANE('',#4879);
#4306=PLANE('',#4880);
#4307=PLANE('',#4881);
#4457=ADVANCED_FACE('',(#516),#4270,.T.);
#4458=ADVANCED_FACE('',(#517),#4271,.F.);
#4459=ADVANCED_FACE('',(#518),#4272,.F.);
#4460=ADVANCED_FACE('',(#519),#4273,.T.);
#4461=ADVANCED_FACE('',(#520),#4274,.T.);
#4462=ADVANCED_FACE('',(#521),#4275,.F.);
#4463=ADVANCED_FACE('',(#522),#4276,.T.);
#4464=ADVANCED_FACE('',(#523),#4277,.F.);
#4465=ADVANCED_FACE('',(#524),#4278,.F.);
#4466=ADVANCED_FACE('',(#525),#4279,.T.);
#4467=ADVANCED_FACE('',(#526),#220,.T.);
#4468=ADVANCED_FACE('',(#527),#221,.T.);
#4469=ADVANCED_FACE('',(#528),#222,.T.);
#4470=ADVANCED_FACE('',(#529),#223,.T.);
#4471=ADVANCED_FACE('',(#530),#4280,.F.);
#4472=ADVANCED_FACE('',(#531),#4281,.F.);
#4473=ADVANCED_FACE('',(#532),#4282,.F.);
#4474=ADVANCED_FACE('',(#533),#4283,.F.);
#4475=ADVANCED_FACE('',(#534),#4284,.F.);
#4476=ADVANCED_FACE('',(#535),#4285,.F.);
#4477=ADVANCED_FACE('',(#536),#4286,.F.);
#4478=ADVANCED_FACE('',(#537),#4287,.F.);
#4479=ADVANCED_FACE('',(#538),#4288,.F.);
#4480=ADVANCED_FACE('',(#539),#4289,.F.);
#4481=ADVANCED_FACE('',(#540),#4290,.F.);
#4482=ADVANCED_FACE('',(#541),#4291,.F.);
#4483=ADVANCED_FACE('',(#542),#4292,.F.);
#4484=ADVANCED_FACE('',(#543),#4293,.F.);
#4485=ADVANCED_FACE('',(#544),#4294,.T.);
#4486=ADVANCED_FACE('',(#545),#4295,.T.);
#4487=ADVANCED_FACE('',(#546),#4296,.T.);
#4488=ADVANCED_FACE('',(#547),#4297,.T.);
#4489=ADVANCED_FACE('',(#548),#4298,.T.);
#4490=ADVANCED_FACE('',(#549),#4299,.T.);
#4491=ADVANCED_FACE('',(#550),#4300,.T.);
#4492=ADVANCED_FACE('',(#551),#4301,.F.);
#4493=ADVANCED_FACE('',(#552),#4302,.F.);
#4494=ADVANCED_FACE('',(#553),#4303,.F.);
#4495=ADVANCED_FACE('',(#554),#4304,.F.);
#4496=ADVANCED_FACE('',(#555),#4305,.F.);
#4497=ADVANCED_FACE('',(#556),#4306,.F.);
#4498=ADVANCED_FACE('',(#557),#4307,.F.);
#4631=CLOSED_SHELL('',(#4457,#4458,#4459,#4460,#4461,#4462,#4463,#4464,
#4465,#4466,#4467,#4468,#4469,#4470,#4471,#4472,#4473,#4474,#4475,#4476,
#4477,#4478,#4479,#4480,#4481,#4482,#4483,#4484,#4485,#4486,#4487,#4488,
#4489,#4490,#4491,#4492,#4493,#4494,#4495,#4496,#4497,#4498));
#4831=AXIS2_PLACEMENT_3D('',#6754,#5457,#5458);
#4832=AXIS2_PLACEMENT_3D('',#6755,#5459,#5460);
#4833=AXIS2_PLACEMENT_3D('',#6764,#5465,#5466);
#4834=AXIS2_PLACEMENT_3D('',#6773,#5471,#5472);
#4835=AXIS2_PLACEMENT_3D('',#6782,#5477,#5478);
#4836=AXIS2_PLACEMENT_3D('',#6791,#5483,#5484);
#4837=AXIS2_PLACEMENT_3D('',#6797,#5487,#5488);
#4838=AXIS2_PLACEMENT_3D('',#6815,#5497,#5498);
#4839=AXIS2_PLACEMENT_3D('',#6832,#5507,#5508);
#4840=AXIS2_PLACEMENT_3D('',#6848,#5517,#5518);
#4841=AXIS2_PLACEMENT_3D('',#6860,#5525,#5526);
#4842=AXIS2_PLACEMENT_3D('',#6877,#5535,#5536);
#4843=AXIS2_PLACEMENT_3D('',#6894,#5545,#5546);
#4844=AXIS2_PLACEMENT_3D('',#6912,#5555,#5556);
#4845=AXIS2_PLACEMENT_3D('',#6928,#5565,#5566);
#4846=AXIS2_PLACEMENT_3D('',#6929,#5567,#5568);
#4847=AXIS2_PLACEMENT_3D('',#6932,#5571,#5572);
#4848=AXIS2_PLACEMENT_3D('',#6935,#5575,#5576);
#4849=AXIS2_PLACEMENT_3D('',#6938,#5579,#5580);
#4850=AXIS2_PLACEMENT_3D('',#6941,#5583,#5584);
#4851=AXIS2_PLACEMENT_3D('',#6942,#5585,#5586);
#4852=AXIS2_PLACEMENT_3D('',#6943,#5587,#5588);
#4853=AXIS2_PLACEMENT_3D('',#6944,#5589,#5590);
#4854=AXIS2_PLACEMENT_3D('',#6945,#5591,#5592);
#4855=AXIS2_PLACEMENT_3D('',#6947,#5594,#5595);
#4856=AXIS2_PLACEMENT_3D('',#6949,#5597,#5598);
#4857=AXIS2_PLACEMENT_3D('',#6951,#5600,#5601);
#4858=AXIS2_PLACEMENT_3D('',#6953,#5603,#5604);
#4859=AXIS2_PLACEMENT_3D('',#6955,#5606,#5607);
#4860=AXIS2_PLACEMENT_3D('',#6957,#5609,#5610);
#4861=AXIS2_PLACEMENT_3D('',#6958,#5611,#5612);
#4862=AXIS2_PLACEMENT_3D('',#6960,#5614,#5615);
#4863=AXIS2_PLACEMENT_3D('',#6962,#5617,#5618);
#4864=AXIS2_PLACEMENT_3D('',#6964,#5620,#5621);
#4865=AXIS2_PLACEMENT_3D('',#6966,#5623,#5624);
#4866=AXIS2_PLACEMENT_3D('',#6968,#5626,#5627);
#4867=AXIS2_PLACEMENT_3D('',#6970,#5629,#5630);
#4868=AXIS2_PLACEMENT_3D('',#6971,#5631,#5632);
#4869=AXIS2_PLACEMENT_3D('',#6973,#5634,#5635);
#4870=AXIS2_PLACEMENT_3D('',#6975,#5637,#5638);
#4871=AXIS2_PLACEMENT_3D('',#6977,#5640,#5641);
#4872=AXIS2_PLACEMENT_3D('',#6979,#5643,#5644);
#4873=AXIS2_PLACEMENT_3D('',#6981,#5646,#5647);
#4874=AXIS2_PLACEMENT_3D('',#6983,#5649,#5650);
#4875=AXIS2_PLACEMENT_3D('',#6984,#5651,#5652);
#4876=AXIS2_PLACEMENT_3D('',#6986,#5654,#5655);
#4877=AXIS2_PLACEMENT_3D('',#6988,#5657,#5658);
#4878=AXIS2_PLACEMENT_3D('',#6990,#5660,#5661);
#4879=AXIS2_PLACEMENT_3D('',#6992,#5663,#5664);
#4880=AXIS2_PLACEMENT_3D('',#6994,#5666,#5667);
#4881=AXIS2_PLACEMENT_3D('',#6996,#5669,#5670);
#5457=DIRECTION('axis',(0.,0.,1.));
#5458=DIRECTION('refdir',(1.,0.,0.));
#5459=DIRECTION('center_axis',(-2.0488859952482E-16,1.,0.));
#5460=DIRECTION('ref_axis',(-1.,-2.0488859952482E-16,0.));
#5461=DIRECTION('',(1.,2.0488859952482E-16,0.));
#5462=DIRECTION('',(0.,0.,1.));
#5463=DIRECTION('',(1.,2.0488859952482E-16,0.));
#5464=DIRECTION('',(0.,0.,-1.));
#5465=DIRECTION('center_axis',(1.,0.,0.));
#5466=DIRECTION('ref_axis',(0.,0.,-1.));
#5467=DIRECTION('',(0.,0.,1.));
#5468=DIRECTION('',(0.,-1.,0.));
#5469=DIRECTION('',(0.,0.,-1.));
#5470=DIRECTION('',(0.,-1.,0.));
#5471=DIRECTION('center_axis',(-1.36592399683213E-16,1.,0.));
#5472=DIRECTION('ref_axis',(-1.,-1.36592399683213E-16,0.));
#5473=DIRECTION('',(0.,0.,1.));
#5474=DIRECTION('',(1.,1.36592399683213E-16,0.));
#5475=DIRECTION('',(0.,0.,-1.));
#5476=DIRECTION('',(1.,1.36592399683213E-16,0.));
#5477=DIRECTION('center_axis',(1.,0.,0.));
#5478=DIRECTION('ref_axis',(0.,0.,-1.));
#5479=DIRECTION('',(0.,-1.,0.));
#5480=DIRECTION('',(0.,0.,1.));
#5481=DIRECTION('',(0.,-1.,0.));
#5482=DIRECTION('',(0.,0.,-1.));
#5483=DIRECTION('center_axis',(0.,0.,1.));
#5484=DIRECTION('ref_axis',(1.,0.,0.));
#5485=DIRECTION('',(-1.,0.,0.));
#5486=DIRECTION('',(0.,-1.,0.));
#5487=DIRECTION('center_axis',(0.,0.,1.));
#5488=DIRECTION('ref_axis',(1.,0.,0.));
#5489=DIRECTION('',(0.,1.,0.));
#5490=DIRECTION('',(-1.,0.,0.));
#5491=DIRECTION('',(0.602092126298966,0.798426622457437,0.));
#5492=DIRECTION('',(1.,0.,0.));
#5493=DIRECTION('',(0.610338133994924,-0.792140998933646,0.));
#5494=DIRECTION('',(-1.,0.,0.));
#5495=DIRECTION('',(0.,-1.,0.));
#5496=DIRECTION('',(1.,2.0488859952482E-16,0.));
#5497=DIRECTION('center_axis',(0.,0.,1.));
#5498=DIRECTION('ref_axis',(1.,0.,0.));
#5499=DIRECTION('',(0.,-1.,0.));
#5500=DIRECTION('',(-1.,0.,0.));
#5501=DIRECTION('',(0.,-1.,0.));
#5502=DIRECTION('',(-0.611447536257502,0.791284974206279,0.));
#5503=DIRECTION('',(0.,1.,0.));
#5504=DIRECTION('',(0.516869211169373,0.85606437757049,0.));
#5505=DIRECTION('',(0.,-1.,0.));
#5506=DIRECTION('',(1.,0.,0.));
#5507=DIRECTION('center_axis',(0.,0.,1.));
#5508=DIRECTION('ref_axis',(1.,0.,0.));
#5509=DIRECTION('',(1.,1.36592399683213E-16,0.));
#5510=DIRECTION('',(0.,1.,0.));
#5511=DIRECTION('',(-1.,0.,0.));
#5512=DIRECTION('',(0.662197771989572,0.749329107116524,0.));
#5513=DIRECTION('',(1.,0.,0.));
#5514=DIRECTION('',(0.729956079204764,-0.683494054423305,0.));
#5515=DIRECTION('',(-1.,0.,0.));
#5516=DIRECTION('',(0.,-1.,0.));
#5517=DIRECTION('center_axis',(0.,0.,1.));
#5518=DIRECTION('ref_axis',(1.,0.,0.));
#5519=DIRECTION('',(1.,0.,0.));
#5520=DIRECTION('',(0.,1.,0.));
#5521=DIRECTION('',(0.507692387525812,-0.861538414493713,0.));
#5522=DIRECTION('',(0.,-1.,0.));
#5523=DIRECTION('',(-0.558176752136098,-0.829722069957644,0.));
#5524=DIRECTION('',(0.,1.,0.));
#5525=DIRECTION('center_axis',(0.,0.,1.));
#5526=DIRECTION('ref_axis',(1.,0.,0.));
#5527=DIRECTION('',(0.,-1.,0.));
#5528=DIRECTION('',(-1.,0.,0.));
#5529=DIRECTION('',(0.,1.,0.));
#5530=DIRECTION('',(-0.558176752136098,-0.829722069957644,0.));
#5531=DIRECTION('',(0.,-1.,0.));
#5532=DIRECTION('',(0.507692387525812,-0.861538414493713,0.));
#5533=DIRECTION('',(0.,1.,0.));
#5534=DIRECTION('',(1.,0.,0.));
#5535=DIRECTION('center_axis',(0.,0.,1.));
#5536=DIRECTION('ref_axis',(1.,0.,0.));
#5537=DIRECTION('',(0.,-1.,0.));
#5538=DIRECTION('',(-1.,0.,0.));
#5539=DIRECTION('',(0.729956079204764,-0.683494054423305,0.));
#5540=DIRECTION('',(1.,0.,0.));
#5541=DIRECTION('',(0.662197771989572,0.749329107116524,0.));
#5542=DIRECTION('',(-1.,0.,0.));
#5543=DIRECTION('',(0.,1.,0.));
#5544=DIRECTION('',(1.,1.36592399683213E-16,0.));
#5545=DIRECTION('center_axis',(0.,0.,1.));
#5546=DIRECTION('ref_axis',(1.,0.,0.));
#5547=DIRECTION('',(1.,0.,0.));
#5548=DIRECTION('',(0.,-1.,0.));
#5549=DIRECTION('',(0.516869211169373,0.85606437757049,0.));
#5550=DIRECTION('',(0.,1.,0.));
#5551=DIRECTION('',(-0.611447536257502,0.791284974206279,0.));
#5552=DIRECTION('',(0.,-1.,0.));
#5553=DIRECTION('',(-1.,0.,0.));
#5554=DIRECTION('',(0.,-1.,0.));
#5555=DIRECTION('center_axis',(0.,0.,1.));
#5556=DIRECTION('ref_axis',(1.,0.,0.));
#5557=DIRECTION('',(1.,2.0488859952482E-16,0.));
#5558=DIRECTION('',(0.,-1.,0.));
#5559=DIRECTION('',(-1.,0.,0.));
#5560=DIRECTION('',(0.610338133994924,-0.792140998933646,0.));
#5561=DIRECTION('',(1.,0.,0.));
#5562=DIRECTION('',(0.602092126298966,0.798426622457437,0.));
#5563=DIRECTION('',(-1.,0.,0.));
#5564=DIRECTION('',(0.,1.,0.));
#5565=DIRECTION('center_axis',(0.,0.,1.));
#5566=DIRECTION('ref_axis',(1.,0.,0.));
#5567=DIRECTION('center_axis',(-2.0488859952482E-16,1.,0.));
#5568=DIRECTION('ref_axis',(-1.,-2.0488859952482E-16,0.));
#5569=DIRECTION('',(0.,0.,1.));
#5570=DIRECTION('',(0.,0.,-1.));
#5571=DIRECTION('center_axis',(1.,0.,0.));
#5572=DIRECTION('ref_axis',(0.,0.,-1.));
#5573=DIRECTION('',(0.,0.,1.));
#5574=DIRECTION('',(0.,0.,-1.));
#5575=DIRECTION('center_axis',(-1.36592399683213E-16,1.,0.));
#5576=DIRECTION('ref_axis',(-1.,-1.36592399683213E-16,0.));
#5577=DIRECTION('',(0.,0.,1.));
#5578=DIRECTION('',(0.,0.,-1.));
#5579=DIRECTION('center_axis',(1.,0.,0.));
#5580=DIRECTION('ref_axis',(0.,0.,-1.));
#5581=DIRECTION('',(0.,0.,1.));
#5582=DIRECTION('',(0.,0.,-1.));
#5583=DIRECTION('center_axis',(0.,0.,1.));
#5584=DIRECTION('ref_axis',(1.,0.,0.));
#5585=DIRECTION('center_axis',(0.,0.,-1.));
#5586=DIRECTION('ref_axis',(-1.,0.,0.));
#5587=DIRECTION('center_axis',(0.,0.,1.));
#5588=DIRECTION('ref_axis',(1.,0.,0.));
#5589=DIRECTION('center_axis',(0.,0.,-1.));
#5590=DIRECTION('ref_axis',(-1.,0.,0.));
#5591=DIRECTION('center_axis',(-1.,0.,0.));
#5592=DIRECTION('ref_axis',(0.,0.,1.));
#5593=DIRECTION('',(0.,0.,1.));
#5594=DIRECTION('center_axis',(0.,1.,0.));
#5595=DIRECTION('ref_axis',(0.,0.,1.));
#5596=DIRECTION('',(0.,0.,1.));
#5597=DIRECTION('center_axis',(-0.792140998933646,-0.610338133994924,0.));
#5598=DIRECTION('ref_axis',(0.610338133994924,-0.792140998933646,0.));
#5599=DIRECTION('',(0.,0.,1.));
#5600=DIRECTION('center_axis',(0.,-1.,0.));
#5601=DIRECTION('ref_axis',(0.,0.,-1.));
#5602=DIRECTION('',(0.,0.,1.));
#5603=DIRECTION('center_axis',(0.798426622457437,-0.602092126298966,0.));
#5604=DIRECTION('ref_axis',(0.602092126298966,0.798426622457437,0.));
#5605=DIRECTION('',(0.,0.,1.));
#5606=DIRECTION('center_axis',(0.,1.,0.));
#5607=DIRECTION('ref_axis',(0.,0.,1.));
#5608=DIRECTION('',(0.,0.,1.));
#5609=DIRECTION('center_axis',(1.,0.,0.));
#5610=DIRECTION('ref_axis',(0.,0.,-1.));
#5611=DIRECTION('center_axis',(0.,-1.,0.));
#5612=DIRECTION('ref_axis',(0.,0.,-1.));
#5613=DIRECTION('',(0.,0.,1.));
#5614=DIRECTION('center_axis',(-1.,0.,0.));
#5615=DIRECTION('ref_axis',(0.,0.,1.));
#5616=DIRECTION('',(0.,0.,1.));
#5617=DIRECTION('center_axis',(0.85606437757049,-0.516869211169373,0.));
#5618=DIRECTION('ref_axis',(0.516869211169373,0.85606437757049,0.));
#5619=DIRECTION('',(0.,0.,1.));
#5620=DIRECTION('center_axis',(1.,0.,0.));
#5621=DIRECTION('ref_axis',(0.,0.,-1.));
#5622=DIRECTION('',(0.,0.,1.));
#5623=DIRECTION('center_axis',(0.791284974206279,0.611447536257502,0.));
#5624=DIRECTION('ref_axis',(-0.611447536257502,0.791284974206279,0.));
#5625=DIRECTION('',(0.,0.,1.));
#5626=DIRECTION('center_axis',(-1.,0.,0.));
#5627=DIRECTION('ref_axis',(0.,0.,1.));
#5628=DIRECTION('',(0.,0.,1.));
#5629=DIRECTION('center_axis',(0.,1.,0.));
#5630=DIRECTION('ref_axis',(0.,0.,1.));
#5631=DIRECTION('center_axis',(1.,0.,0.));
#5632=DIRECTION('ref_axis',(0.,0.,-1.));
#5633=DIRECTION('',(0.,0.,1.));
#5634=DIRECTION('center_axis',(-1.,0.,0.));
#5635=DIRECTION('ref_axis',(0.,0.,1.));
#5636=DIRECTION('',(0.,0.,1.));
#5637=DIRECTION('center_axis',(0.,1.,0.));
#5638=DIRECTION('ref_axis',(0.,0.,1.));
#5639=DIRECTION('',(0.,0.,1.));
#5640=DIRECTION('center_axis',(-0.683494054423305,-0.729956079204764,0.));
#5641=DIRECTION('ref_axis',(0.729956079204764,-0.683494054423305,0.));
#5642=DIRECTION('',(0.,0.,1.));
#5643=DIRECTION('center_axis',(0.,-1.,0.));
#5644=DIRECTION('ref_axis',(0.,0.,-1.));
#5645=DIRECTION('',(0.,0.,1.));
#5646=DIRECTION('center_axis',(0.749329107116524,-0.662197771989572,0.));
#5647=DIRECTION('ref_axis',(0.662197771989572,0.749329107116524,0.));
#5648=DIRECTION('',(0.,0.,1.));
#5649=DIRECTION('center_axis',(0.,1.,0.));
#5650=DIRECTION('ref_axis',(0.,0.,1.));
#5651=DIRECTION('center_axis',(0.,1.,0.));
#5652=DIRECTION('ref_axis',(0.,0.,1.));
#5653=DIRECTION('',(0.,0.,1.));
#5654=DIRECTION('center_axis',(1.,0.,0.));
#5655=DIRECTION('ref_axis',(0.,0.,-1.));
#5656=DIRECTION('',(0.,0.,1.));
#5657=DIRECTION('center_axis',(-0.829722069957644,0.558176752136098,0.));
#5658=DIRECTION('ref_axis',(-0.558176752136098,-0.829722069957644,0.));
#5659=DIRECTION('',(0.,0.,1.));
#5660=DIRECTION('center_axis',(-1.,0.,0.));
#5661=DIRECTION('ref_axis',(0.,0.,1.));
#5662=DIRECTION('',(0.,0.,1.));
#5663=DIRECTION('center_axis',(-0.861538414493713,-0.507692387525812,0.));
#5664=DIRECTION('ref_axis',(0.507692387525812,-0.861538414493713,0.));
#5665=DIRECTION('',(0.,0.,1.));
#5666=DIRECTION('center_axis',(1.,0.,0.));
#5667=DIRECTION('ref_axis',(0.,0.,-1.));
#5668=DIRECTION('',(0.,0.,1.));
#5669=DIRECTION('center_axis',(0.,-1.,0.));
#5670=DIRECTION('ref_axis',(0.,0.,-1.));
#6754=CARTESIAN_POINT('',(0.,0.,0.));
#6755=CARTESIAN_POINT('Origin',(1.7347234759768E-18,0.0127,0.215));
#6756=CARTESIAN_POINT('',(0.00344930659048259,0.0127,0.));
#6757=CARTESIAN_POINT('',(0.0097,0.0127,0.));
#6758=CARTESIAN_POINT('',(1.7347234759768E-18,0.0127,0.));
#6759=CARTESIAN_POINT('',(0.00344930659048259,0.0127,0.215));
#6760=CARTESIAN_POINT('',(0.00344930659048259,0.0127,-0.015));
#6761=CARTESIAN_POINT('',(0.0097,0.0127,0.215));
#6762=CARTESIAN_POINT('',(1.7347234759768E-18,0.0127,0.215));
#6763=CARTESIAN_POINT('',(0.0097,0.0127,0.215));
#6764=CARTESIAN_POINT('Origin',(-0.0127,-3.46944695195361E-18,0.215));
#6765=CARTESIAN_POINT('',(-0.0127,-0.00262824492529034,0.));
#6766=CARTESIAN_POINT('',(-0.0127,-0.00262824492529034,0.215));
#6767=CARTESIAN_POINT('',(-0.0127,-0.00262824492529034,-0.015));
#6768=CARTESIAN_POINT('',(-0.0127,-0.0097,0.));
#6769=CARTESIAN_POINT('',(-0.0127,-3.46944695195361E-18,0.));
#6770=CARTESIAN_POINT('',(-0.0127,-0.0097,0.215));
#6771=CARTESIAN_POINT('',(-0.0127,-0.0097,0.215));
#6772=CARTESIAN_POINT('',(-0.0127,-3.46944695195361E-18,0.215));
#6773=CARTESIAN_POINT('Origin',(1.7347234759768E-18,-0.0127,0.215));
#6774=CARTESIAN_POINT('',(0.00344930659048259,-0.0127,0.));
#6775=CARTESIAN_POINT('',(0.00344930659048259,-0.0127,0.215));
#6776=CARTESIAN_POINT('',(0.00344930659048259,-0.0127,-0.015));
#6777=CARTESIAN_POINT('',(0.0097,-0.0127,0.));
#6778=CARTESIAN_POINT('',(1.7347234759768E-18,-0.0127,0.));
#6779=CARTESIAN_POINT('',(0.0097,-0.0127,0.215));
#6780=CARTESIAN_POINT('',(0.0097,-0.0127,0.215));
#6781=CARTESIAN_POINT('',(1.7347234759768E-18,-0.0127,0.215));
#6782=CARTESIAN_POINT('Origin',(0.0127,1.7347234759768E-18,0.215));
#6783=CARTESIAN_POINT('',(0.0127,-0.00192708557005971,0.));
#6784=CARTESIAN_POINT('',(0.0127,-0.0097,0.));
#6785=CARTESIAN_POINT('',(0.0127,1.7347234759768E-18,0.));
#6786=CARTESIAN_POINT('',(0.0127,-0.00192708557005971,0.215));
#6787=CARTESIAN_POINT('',(0.0127,-0.00192708557005971,-0.015));
#6788=CARTESIAN_POINT('',(0.0127,-0.0097,0.215));
#6789=CARTESIAN_POINT('',(0.0127,1.7347234759768E-18,0.215));
#6790=CARTESIAN_POINT('',(0.0127,-0.0097,0.));
#6791=CARTESIAN_POINT('Origin',(0.,0.,0.215));
#6792=CARTESIAN_POINT('',(0.0127,0.00368218845687806,0.215));
#6793=CARTESIAN_POINT('',(0.0110062453895807,0.00368218845687806,0.215));
#6794=CARTESIAN_POINT('',(0.0118531226947904,0.00368218845687806,0.215));
#6795=CARTESIAN_POINT('',(0.0127,0.0097,0.215));
#6796=CARTESIAN_POINT('',(0.0127,1.7347234759768E-18,0.215));
#6797=CARTESIAN_POINT('Origin',(0.0097,0.0097,0.215));
#6798=CARTESIAN_POINT('',(0.00344930659048259,0.0110833141952753,0.215));
#6799=CARTESIAN_POINT('',(0.00344930659048259,0.0118916570976376,0.215));
#6800=CARTESIAN_POINT('',(0.0082016084343195,0.0110833141952753,0.215));
#6801=CARTESIAN_POINT('',(0.00582545751240104,0.0110833141952753,0.215));
#6802=CARTESIAN_POINT('',(0.00461790570989251,0.00633101211860776,0.215));
#6803=CARTESIAN_POINT('',(0.006409757072106,0.00870716315694153,0.215));
#6804=CARTESIAN_POINT('',(-0.00402972521260381,0.00633101211860776,0.215));
#6805=CARTESIAN_POINT('',(0.000294090248644352,0.00633101211860776,0.215));
#6806=CARTESIAN_POINT('',(-0.00769133493304253,0.0110833141952753,0.215));
#6807=CARTESIAN_POINT('',(-0.00586053007282317,0.00870716315694153,0.215));
#6808=CARTESIAN_POINT('',(-0.00332856620661914,0.0110833141952753,0.215));
#6809=CARTESIAN_POINT('',(-0.00550995056983084,0.0110833141952753,0.215));
#6810=CARTESIAN_POINT('',(-0.00332856620661914,0.0127,0.215));
#6811=CARTESIAN_POINT('',(-0.00332856620661914,0.0118916570976376,0.215));
#6812=CARTESIAN_POINT('',(-0.0097,0.0127,0.215));
#6813=CARTESIAN_POINT('',(1.7347234759768E-18,0.0127,0.215));
#6814=CARTESIAN_POINT('',(-0.0127,0.0097,0.215));
#6815=CARTESIAN_POINT('Origin',(-0.0097,0.0097,0.215));
#6816=CARTESIAN_POINT('',(-0.0127,0.00368218845687806,0.215));
#6817=CARTESIAN_POINT('',(-0.0127,-3.46944695195361E-18,0.215));
#6818=CARTESIAN_POINT('',(-0.0108075980097055,0.00368218845687806,0.215));
#6819=CARTESIAN_POINT('',(-0.0117537990048528,0.00368218845687806,0.215));
#6820=CARTESIAN_POINT('',(-0.0108075980097055,0.00711007788777351,0.215));
#6821=CARTESIAN_POINT('',(-0.0108075980097055,0.00539613317232579,0.215));
#6822=CARTESIAN_POINT('',(-0.00815877411514521,0.00368218845687806,0.215));
#6823=CARTESIAN_POINT('',(-0.00948318606242537,0.00539613317232579,0.215));
#6824=CARTESIAN_POINT('',(-0.00815877411514521,-0.00403056340292096,0.215));
#6825=CARTESIAN_POINT('',(-0.00815877411514521,-0.000174187473021447,0.215));
#6826=CARTESIAN_POINT('',(-0.0106517849490046,-0.00815961137413979,0.215));
#6827=CARTESIAN_POINT('',(-0.00940527953207493,-0.00609508738853037,0.215));
#6828=CARTESIAN_POINT('',(-0.0106517849490046,-0.00262824492529034,0.215));
#6829=CARTESIAN_POINT('',(-0.0106517849490046,-0.00539392814971507,0.215));
#6830=CARTESIAN_POINT('',(-0.0116758924745023,-0.00262824492529034,0.215));
#6831=CARTESIAN_POINT('',(-0.0097,-0.0127,0.215));
#6832=CARTESIAN_POINT('Origin',(-0.0097,-0.0097,0.215));
#6833=CARTESIAN_POINT('',(-0.00332856620661914,-0.0127,0.215));
#6834=CARTESIAN_POINT('',(1.7347234759768E-18,-0.0127,0.215));
#6835=CARTESIAN_POINT('',(-0.00332856620661914,-0.0104968100786209,0.215));
#6836=CARTESIAN_POINT('',(-0.00332856620661914,-0.0115984050393105,0.215));
#6837=CARTESIAN_POINT('',(-0.00815877411514521,-0.0104968100786209,0.215));
#6838=CARTESIAN_POINT('',(-0.00574367016088218,-0.0104968100786209,0.215));
#6839=CARTESIAN_POINT('',(-0.00519832409918308,-0.00714682694524527,0.215));
#6840=CARTESIAN_POINT('',(-0.00667854910716415,-0.00882181851193309,0.215));
#6841=CARTESIAN_POINT('',(0.00344930659048259,-0.00714682694524527,0.215));
#6842=CARTESIAN_POINT('',(-0.000874508754350245,-0.00714682694524527,0.215));
#6843=CARTESIAN_POINT('',(0.00617603724822402,-0.0097,0.215));
#6844=CARTESIAN_POINT('',(0.00481267191935331,-0.00842341347262263,0.215));
#6845=CARTESIAN_POINT('',(0.00344930659048259,-0.0097,0.215));
#6846=CARTESIAN_POINT('',(0.00481267191935331,-0.0097,0.215));
#6847=CARTESIAN_POINT('',(0.00344930659048259,-0.0112,0.215));
#6848=CARTESIAN_POINT('Origin',(0.0097,-0.0097,0.215));
#6849=CARTESIAN_POINT('',(0.0106946192681789,-0.00192708557005971,0.215));
#6850=CARTESIAN_POINT('',(0.0116973096340895,-0.00192708557005971,0.215));
#6851=CARTESIAN_POINT('',(0.0106946192681789,-0.00800379924476147,0.215));
#6852=CARTESIAN_POINT('',(0.0106946192681789,-0.00496544240741059,0.215));
#6853=CARTESIAN_POINT('',(0.00812370143830776,-0.00364103051833809,0.215));
#6854=CARTESIAN_POINT('',(0.00940916035324335,-0.00582241488154978,0.215));
#6855=CARTESIAN_POINT('',(0.00812370143830776,0.00477288058027625,0.215));
#6856=CARTESIAN_POINT('',(0.00812370143830776,0.000565925030969083,0.215));
#6857=CARTESIAN_POINT('',(0.0110062453895807,0.00905774254351854,0.215));
#6858=CARTESIAN_POINT('',(0.00956497341394424,0.0069153115618974,0.215));
#6859=CARTESIAN_POINT('',(0.0110062453895807,0.00636996550019831,0.215));
#6860=CARTESIAN_POINT('Origin',(0.,0.,0.));
#6861=CARTESIAN_POINT('',(0.0127,0.0097,0.));
#6862=CARTESIAN_POINT('',(0.0127,0.00368218845687806,0.));
#6863=CARTESIAN_POINT('',(0.0127,1.7347234759768E-18,0.));
#6864=CARTESIAN_POINT('',(0.0110062453895807,0.00368218845687806,0.));
#6865=CARTESIAN_POINT('',(0.,0.00368218845687806,0.));
#6866=CARTESIAN_POINT('',(0.0110062453895807,0.00905774254351854,0.));
#6867=CARTESIAN_POINT('',(0.0110062453895807,0.,0.));
#6868=CARTESIAN_POINT('',(0.00812370143830776,0.00477288058027625,0.));
#6869=CARTESIAN_POINT('',(0.00338219888858266,-0.00227529778833503,0.));
#6870=CARTESIAN_POINT('',(0.00812370143830776,-0.00364103051833809,0.));
#6871=CARTESIAN_POINT('',(0.00812370143830776,0.,0.));
#6872=CARTESIAN_POINT('',(0.0106946192681789,-0.00800379924476147,0.));
#6873=CARTESIAN_POINT('',(0.00443723073130199,0.0026147972348992,0.));
#6874=CARTESIAN_POINT('',(0.0106946192681789,-0.00192708557005971,0.));
#6875=CARTESIAN_POINT('',(0.0106946192681789,0.,0.));
#6876=CARTESIAN_POINT('',(0.,-0.00192708557005971,0.));
#6877=CARTESIAN_POINT('Origin',(0.0097,-0.0097,0.));
#6878=CARTESIAN_POINT('',(0.00344930659048259,-0.0097,0.));
#6879=CARTESIAN_POINT('',(0.00344930659048259,0.,0.));
#6880=CARTESIAN_POINT('',(0.00617603724822402,-0.0097,0.));
#6881=CARTESIAN_POINT('',(0.,-0.0097,0.));
#6882=CARTESIAN_POINT('',(0.00344930659048259,-0.00714682694524527,0.));
#6883=CARTESIAN_POINT('',(-0.00195430718805409,-0.00208715555507985,0.));
#6884=CARTESIAN_POINT('',(-0.00519832409918308,-0.00714682694524527,0.));
#6885=CARTESIAN_POINT('',(0.,-0.00714682694524527,0.));
#6886=CARTESIAN_POINT('',(-0.00815877411514521,-0.0104968100786209,0.));
#6887=CARTESIAN_POINT('',(0.000627456216075237,-0.000554496154439945,0.));
#6888=CARTESIAN_POINT('',(-0.00332856620661914,-0.0104968100786209,0.));
#6889=CARTESIAN_POINT('',(0.,-0.0104968100786209,0.));
#6890=CARTESIAN_POINT('',(-0.00332856620661914,-0.0127,0.));
#6891=CARTESIAN_POINT('',(-0.00332856620661914,0.,0.));
#6892=CARTESIAN_POINT('',(-0.0097,-0.0127,0.));
#6893=CARTESIAN_POINT('',(1.7347234759768E-18,-0.0127,0.));
#6894=CARTESIAN_POINT('Origin',(-0.0097,-0.0097,0.));
#6895=CARTESIAN_POINT('',(-0.0106517849490046,-0.00262824492529034,0.));
#6896=CARTESIAN_POINT('',(0.,-0.00262824492529034,0.));
#6897=CARTESIAN_POINT('',(-0.0106517849490046,-0.00815961137413979,0.));
#6898=CARTESIAN_POINT('',(-0.0106517849490046,0.,0.));
#6899=CARTESIAN_POINT('',(-0.00815877411514521,-0.00403056340292096,0.));
#6900=CARTESIAN_POINT('',(-0.00419570998972095,0.00253325961166274,0.));
#6901=CARTESIAN_POINT('',(-0.00815877411514521,0.00368218845687806,0.));
#6902=CARTESIAN_POINT('',(-0.00815877411514521,0.,0.));
#6903=CARTESIAN_POINT('',(-0.0108075980097055,0.00711007788777351,0.));
#6904=CARTESIAN_POINT('',(-0.0033269183513521,-0.00257080078047055,0.));
#6905=CARTESIAN_POINT('',(-0.0108075980097055,0.00368218845687806,0.));
#6906=CARTESIAN_POINT('',(-0.0108075980097055,0.,0.));
#6907=CARTESIAN_POINT('',(-0.0127,0.00368218845687806,0.));
#6908=CARTESIAN_POINT('',(0.,0.00368218845687806,0.));
#6909=CARTESIAN_POINT('',(-0.0127,0.0097,0.));
#6910=CARTESIAN_POINT('',(-0.0127,-3.46944695195361E-18,0.));
#6911=CARTESIAN_POINT('',(-0.0097,0.0127,0.));
#6912=CARTESIAN_POINT('Origin',(-0.0097,0.0097,0.));
#6913=CARTESIAN_POINT('',(-0.00332856620661914,0.0127,0.));
#6914=CARTESIAN_POINT('',(1.7347234759768E-18,0.0127,0.));
#6915=CARTESIAN_POINT('',(-0.00332856620661914,0.0110833141952753,0.));
#6916=CARTESIAN_POINT('',(-0.00332856620661914,0.,0.));
#6917=CARTESIAN_POINT('',(-0.00769133493304253,0.0110833141952753,0.));
#6918=CARTESIAN_POINT('',(0.,0.0110833141952753,0.));
#6919=CARTESIAN_POINT('',(-0.00402972521260381,0.00633101211860776,0.));
#6920=CARTESIAN_POINT('',(0.000532277217295219,0.000410115224447797,0.));
#6921=CARTESIAN_POINT('',(0.00461790570989251,0.00633101211860776,0.));
#6922=CARTESIAN_POINT('',(0.,0.00633101211860776,0.));
#6923=CARTESIAN_POINT('',(0.0082016084343195,0.0110833141952753,0.));
#6924=CARTESIAN_POINT('',(-9.96386038842768E-5,7.51372977638188E-5,0.));
#6925=CARTESIAN_POINT('',(0.00344930659048259,0.0110833141952753,0.));
#6926=CARTESIAN_POINT('',(0.,0.0110833141952753,0.));
#6927=CARTESIAN_POINT('',(0.00344930659048259,0.,0.));
#6928=CARTESIAN_POINT('Origin',(0.0097,0.0097,0.));
#6929=CARTESIAN_POINT('Origin',(1.7347234759768E-18,0.0127,0.215));
#6930=CARTESIAN_POINT('',(-0.00332856620661914,0.0127,-0.015));
#6931=CARTESIAN_POINT('',(-0.0097,0.0127,0.215));
#6932=CARTESIAN_POINT('Origin',(-0.0127,-3.46944695195361E-18,0.215));
#6933=CARTESIAN_POINT('',(-0.0127,0.00368218845687806,-0.015));
#6934=CARTESIAN_POINT('',(-0.0127,0.0097,0.));
#6935=CARTESIAN_POINT('Origin',(1.7347234759768E-18,-0.0127,0.215));
#6936=CARTESIAN_POINT('',(-0.00332856620661914,-0.0127,-0.015));
#6937=CARTESIAN_POINT('',(-0.0097,-0.0127,0.215));
#6938=CARTESIAN_POINT('Origin',(0.0127,1.7347234759768E-18,0.215));
#6939=CARTESIAN_POINT('',(0.0127,0.00368218845687806,-0.015));
#6940=CARTESIAN_POINT('',(0.0127,0.0097,0.215));
#6941=CARTESIAN_POINT('Origin',(-0.0097,0.0097,0.215));
#6942=CARTESIAN_POINT('Origin',(-0.0097,-0.0097,0.215));
#6943=CARTESIAN_POINT('Origin',(0.0097,-0.0097,0.215));
#6944=CARTESIAN_POINT('Origin',(0.0097,0.0097,0.215));
#6945=CARTESIAN_POINT('Origin',(-0.00332856620661914,0.0118916570976376,
-0.015));
#6946=CARTESIAN_POINT('',(-0.00332856620661914,0.0110833141952753,-0.015));
#6947=CARTESIAN_POINT('Origin',(-0.00550995056983084,0.0110833141952753,
-0.015));
#6948=CARTESIAN_POINT('',(-0.00769133493304253,0.0110833141952753,-0.015));
#6949=CARTESIAN_POINT('Origin',(-0.00586053007282317,0.00870716315694153,
-0.015));
#6950=CARTESIAN_POINT('',(-0.00402972521260381,0.00633101211860776,-0.015));
#6951=CARTESIAN_POINT('Origin',(0.000294090248644352,0.00633101211860776,
-0.015));
#6952=CARTESIAN_POINT('',(0.00461790570989251,0.00633101211860776,-0.015));
#6953=CARTESIAN_POINT('Origin',(0.006409757072106,0.00870716315694153,-0.015));
#6954=CARTESIAN_POINT('',(0.0082016084343195,0.0110833141952753,-0.015));
#6955=CARTESIAN_POINT('Origin',(0.00582545751240104,0.0110833141952753,
-0.015));
#6956=CARTESIAN_POINT('',(0.00344930659048259,0.0110833141952753,-0.015));
#6957=CARTESIAN_POINT('Origin',(0.00344930659048259,0.0118916570976376,
-0.015));
#6958=CARTESIAN_POINT('Origin',(-0.0116758924745023,-0.00262824492529034,
-0.015));
#6959=CARTESIAN_POINT('',(-0.0106517849490046,-0.00262824492529034,-0.015));
#6960=CARTESIAN_POINT('Origin',(-0.0106517849490046,-0.00539392814971507,
-0.015));
#6961=CARTESIAN_POINT('',(-0.0106517849490046,-0.00815961137413979,-0.015));
#6962=CARTESIAN_POINT('Origin',(-0.00940527953207493,-0.00609508738853037,
-0.015));
#6963=CARTESIAN_POINT('',(-0.00815877411514521,-0.00403056340292096,-0.015));
#6964=CARTESIAN_POINT('Origin',(-0.00815877411514521,-0.000174187473021447,
-0.015));
#6965=CARTESIAN_POINT('',(-0.00815877411514521,0.00368218845687806,-0.015));
#6966=CARTESIAN_POINT('Origin',(-0.00948318606242537,0.00539613317232579,
-0.015));
#6967=CARTESIAN_POINT('',(-0.0108075980097055,0.00711007788777351,-0.015));
#6968=CARTESIAN_POINT('Origin',(-0.0108075980097055,0.00539613317232579,
-0.015));
#6969=CARTESIAN_POINT('',(-0.0108075980097055,0.00368218845687806,-0.015));
#6970=CARTESIAN_POINT('Origin',(-0.0117537990048528,0.00368218845687806,
-0.015));
#6971=CARTESIAN_POINT('Origin',(-0.00332856620661914,-0.0115984050393105,
-0.015));
#6972=CARTESIAN_POINT('',(-0.00332856620661914,-0.0104968100786209,-0.015));
#6973=CARTESIAN_POINT('Origin',(0.00344930659048259,-0.0112,-0.015));
#6974=CARTESIAN_POINT('',(0.00344930659048259,-0.0097,-0.015));
#6975=CARTESIAN_POINT('Origin',(0.00481267191935331,-0.0097,-0.015));
#6976=CARTESIAN_POINT('',(0.00617603724822402,-0.0097,-0.015));
#6977=CARTESIAN_POINT('Origin',(0.00481267191935331,-0.00842341347262263,
-0.015));
#6978=CARTESIAN_POINT('',(0.00344930659048259,-0.00714682694524527,-0.015));
#6979=CARTESIAN_POINT('Origin',(-0.000874508754350245,-0.00714682694524527,
-0.015));
#6980=CARTESIAN_POINT('',(-0.00519832409918308,-0.00714682694524527,-0.015));
#6981=CARTESIAN_POINT('Origin',(-0.00667854910716415,-0.00882181851193309,
-0.015));
#6982=CARTESIAN_POINT('',(-0.00815877411514521,-0.0104968100786209,-0.015));
#6983=CARTESIAN_POINT('Origin',(-0.00574367016088218,-0.0104968100786209,
-0.015));
#6984=CARTESIAN_POINT('Origin',(0.0118531226947904,0.00368218845687806,
-0.015));
#6985=CARTESIAN_POINT('',(0.0110062453895807,0.00368218845687806,-0.015));
#6986=CARTESIAN_POINT('Origin',(0.0110062453895807,0.00636996550019831,
-0.015));
#6987=CARTESIAN_POINT('',(0.0110062453895807,0.00905774254351854,-0.015));
#6988=CARTESIAN_POINT('Origin',(0.00956497341394424,0.0069153115618974,
-0.015));
#6989=CARTESIAN_POINT('',(0.00812370143830776,0.00477288058027625,-0.015));
#6990=CARTESIAN_POINT('Origin',(0.00812370143830776,0.000565925030969083,
-0.015));
#6991=CARTESIAN_POINT('',(0.00812370143830776,-0.00364103051833809,-0.015));
#6992=CARTESIAN_POINT('Origin',(0.00940916035324335,-0.00582241488154978,
-0.015));
#6993=CARTESIAN_POINT('',(0.0106946192681789,-0.00800379924476147,-0.015));
#6994=CARTESIAN_POINT('Origin',(0.0106946192681789,-0.00496544240741059,
-0.015));
#6995=CARTESIAN_POINT('',(0.0106946192681789,-0.00192708557005971,-0.015));
#6996=CARTESIAN_POINT('Origin',(0.0116973096340895,-0.00192708557005971,
-0.015));
#7741=UNCERTAINTY_MEASURE_WITH_UNIT(LENGTH_MEASURE(1.E-5),#7757,
'DISTANCE_ACCURACY_VALUE',
'Maximum model space distance between geometric entities at asserted c
onnectivities');
#7745=UNCERTAINTY_MEASURE_WITH_UNIT(LENGTH_MEASURE(1.E-5),#7757,
'DISTANCE_ACCURACY_VALUE',
'Maximum model space distance between geometric entities at asserted c
onnectivities');
#7752=(
GEOMETRIC_REPRESENTATION_CONTEXT(3)
GLOBAL_UNCERTAINTY_ASSIGNED_CONTEXT((#7741))
GLOBAL_UNIT_ASSIGNED_CONTEXT((#7757,#7758,#7759))
REPRESENTATION_CONTEXT('','3D')
);
#7756=(
GEOMETRIC_REPRESENTATION_CONTEXT(3)
GLOBAL_UNCERTAINTY_ASSIGNED_CONTEXT((#7745))
GLOBAL_UNIT_ASSIGNED_CONTEXT((#7757,#7758,#7759))
REPRESENTATION_CONTEXT('','3D')
);
#7757=(
LENGTH_UNIT()
NAMED_UNIT(*)
SI_UNIT($,.METRE.)
);
#7758=(
NAMED_UNIT(*)
PLANE_ANGLE_UNIT()
SI_UNIT($,.RADIAN.)
);
#7759=(
NAMED_UNIT(*)
SI_UNIT($,.STERADIAN.)
SOLID_ANGLE_UNIT()
);
#7766=SHAPE_DEFINITION_REPRESENTATION(#7776,#7824);
#7776=PRODUCT_DEFINITION_SHAPE('',$,#7835);
#7824=SHAPE_REPRESENTATION('',(#4831),#7752);
#7828=PRODUCT_DEFINITION_CONTEXT('part definition',#7860,'design');
#7835=PRODUCT_DEFINITION('1010 Aluminum Extrusion',
'1010 Aluminum Extrusion',#7845,#7828);
#7845=PRODUCT_DEFINITION_FORMATION('',$,#7868);
#7860=APPLICATION_CONTEXT(
'Core Data for Automotive Mechanical Design Process');
#7861=PRODUCT_CONTEXT('part definition',#7860,'mechanical');
#7868=PRODUCT('1010 Aluminum Extrusion','1010 Aluminum Extrusion',
'LEGAL AND USAGE DISCLAIMER: this Data/Model is provided \X2\201C\X0\A
S IS\X2\201D\X0\ for informational and representational only. It is a 
geometric approximation and is NOT engineered, certified, or guarantee
d for dimensional accuracy, exact tolerances, or production-level prec
ision. Vendor disclaims all implied warranties including fitness for a
 particular purpose. DO NOT USE FOR DIRECT PHYSICAL MANUFACTURING, AUT
OMATED PRODUCTION, OR SAFETY-CRITICAL SYSTEMS without independent engi
neering verification and resolution of any design discrepancies.',(#7861));
#7875=PRESENTATION_STYLE_ASSIGNMENT((#7882));
#7882=SURFACE_STYLE_USAGE(.BOTH.,#7889);
#7889=SURFACE_SIDE_STYLE('',(#7896));
#7896=SURFACE_STYLE_FILL_AREA(#7903);
#7903=FILL_AREA_STYLE('Opaque(25,25,25)',(#7910));
#7910=FILL_AREA_STYLE_COLOUR('Opaque(25,25,25)',#7917);
#7917=COLOUR_RGB('Opaque(25,25,25)',0.0980392156862745,0.0980392156862745,
0.0980392156862745);
ENDSEC;
END-ISO-10303-21;
